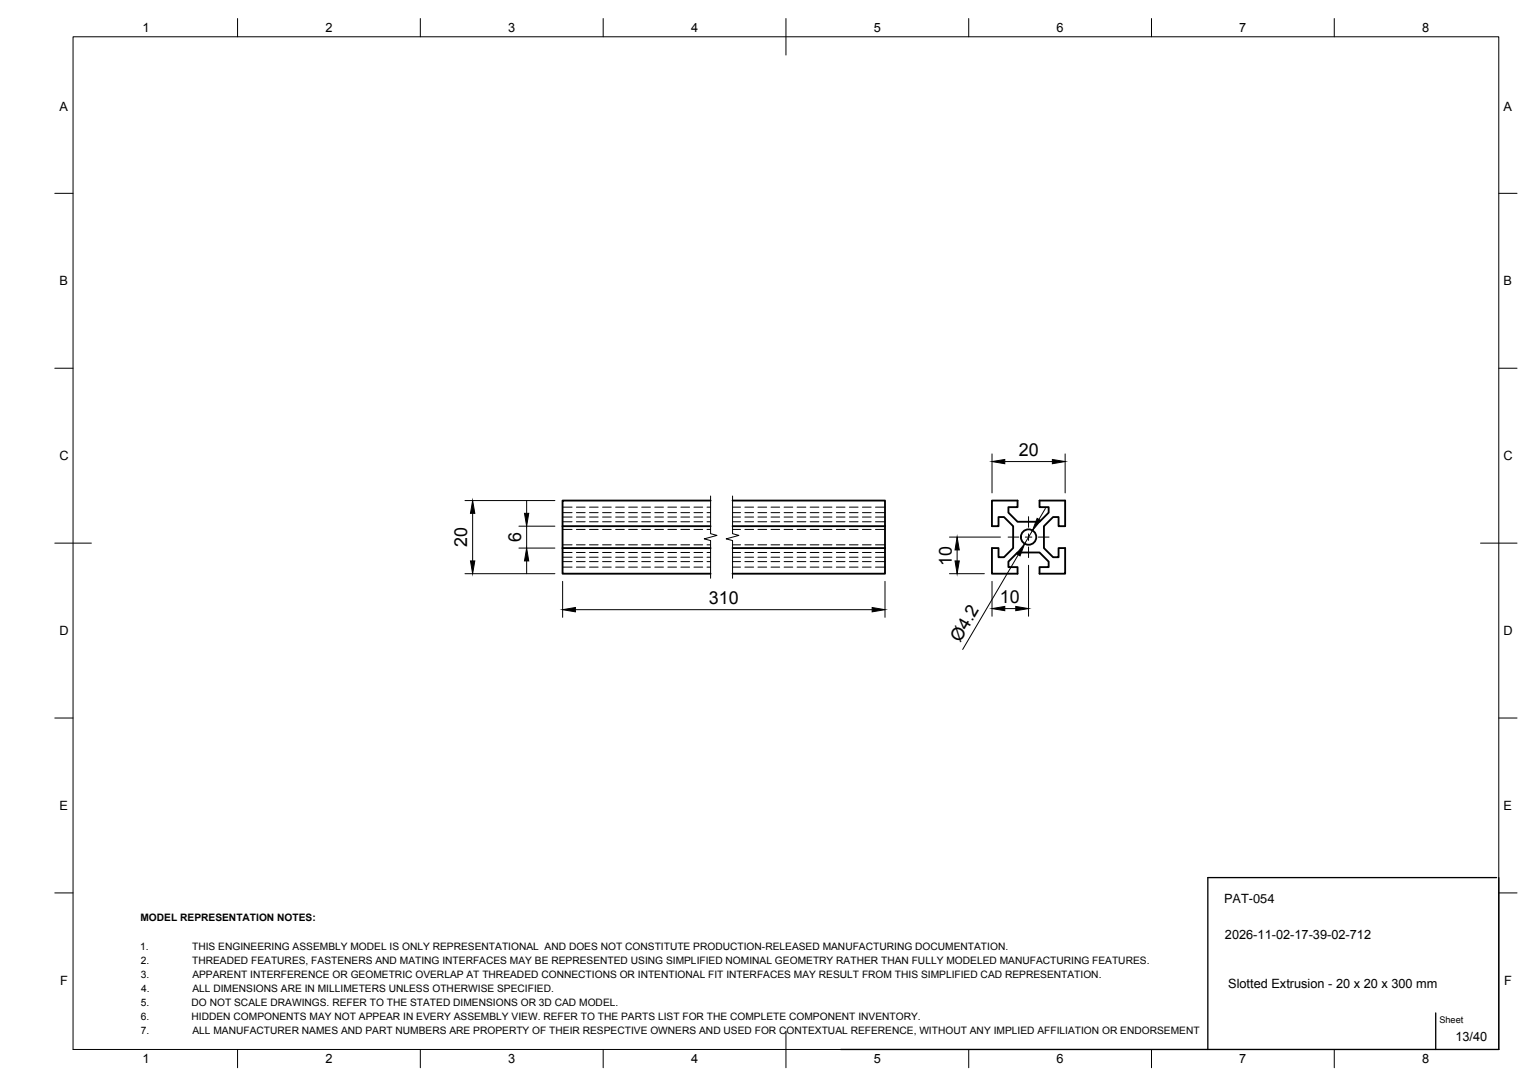
ISO-10303-21;
HEADER;
/* Generated by software containing ST-Developer
 * from STEP Tools, Inc. (www.steptools.com) 
 */

FILE_DESCRIPTION(
/* description */ ('PAT-054'),
/* implementation_level */ '2;1');

FILE_NAME(
/* name */ 'Slotted Extrusion - 20 x 20 x 300 mm.step',
/* time_stamp */ '2026-10-29T16:38:13-07:00',
/* author */ (''),
/* organization */ (''),
/* preprocessor_version */ 'ST-DEVELOPER v20.2',
/* originating_system */ 'Autodesk Translation Framework v15.17.0.0',
/* authorisation */ '');

FILE_SCHEMA (('AUTOMOTIVE_DESIGN { 1 0 10303 214 3 1 1 }'));
ENDSEC;

DATA;
#10=MECHANICAL_DESIGN_GEOMETRIC_PRESENTATION_REPRESENTATION('',(#933),#33981);
#830=SHAPE_REPRESENTATION_RELATIONSHIP('SRR','None',#34205,#874);
#874=ADVANCED_BREP_SHAPE_REPRESENTATION('',(#992),#33953);
#933=STYLED_ITEM('',(#34531),#992);
#992=MANIFOLD_SOLID_BREP('Body1',#13044);
#1146=FACE_BOUND('',#2730,.T.);
#1147=FACE_BOUND('',#2732,.T.);
#1344=PLANE('',#14134);
#1345=PLANE('',#14135);
#1346=PLANE('',#14136);
#1347=PLANE('',#14137);
#1348=PLANE('',#14138);
#1349=PLANE('',#14139);
#1350=PLANE('',#14140);
#1351=PLANE('',#14141);
#1352=PLANE('',#14142);
#1353=PLANE('',#14143);
#1354=PLANE('',#14144);
#1355=PLANE('',#14145);
#1356=PLANE('',#14146);
#1357=PLANE('',#14147);
#1358=PLANE('',#14148);
#1359=PLANE('',#14149);
#1360=PLANE('',#14150);
#1361=PLANE('',#14151);
#1362=PLANE('',#14152);
#1363=PLANE('',#14153);
#1364=PLANE('',#14154);
#1365=PLANE('',#14155);
#1366=PLANE('',#14156);
#1367=PLANE('',#14157);
#1368=PLANE('',#14158);
#1369=PLANE('',#14159);
#1370=PLANE('',#14160);
#1371=PLANE('',#14161);
#1372=PLANE('',#14162);
#1373=PLANE('',#14163);
#1374=PLANE('',#14164);
#1375=PLANE('',#14165);
#1376=PLANE('',#14166);
#1377=PLANE('',#14167);
#1378=PLANE('',#14168);
#1379=PLANE('',#14169);
#1380=PLANE('',#14173);
#1381=PLANE('',#14174);
#1382=PLANE('',#14175);
#1383=PLANE('',#14176);
#1384=PLANE('',#14177);
#1385=PLANE('',#14178);
#1386=PLANE('',#14179);
#1387=PLANE('',#14180);
#1388=PLANE('',#14181);
#1389=PLANE('',#14182);
#1827=FACE_OUTER_BOUND('',#2684,.T.);
#1828=FACE_OUTER_BOUND('',#2685,.T.);
#1829=FACE_OUTER_BOUND('',#2686,.T.);
#1830=FACE_OUTER_BOUND('',#2687,.T.);
#1831=FACE_OUTER_BOUND('',#2688,.T.);
#1832=FACE_OUTER_BOUND('',#2689,.T.);
#1833=FACE_OUTER_BOUND('',#2690,.T.);
#1834=FACE_OUTER_BOUND('',#2691,.T.);
#1835=FACE_OUTER_BOUND('',#2692,.T.);
#1836=FACE_OUTER_BOUND('',#2693,.T.);
#1837=FACE_OUTER_BOUND('',#2694,.T.);
#1838=FACE_OUTER_BOUND('',#2695,.T.);
#1839=FACE_OUTER_BOUND('',#2696,.T.);
#1840=FACE_OUTER_BOUND('',#2697,.T.);
#1841=FACE_OUTER_BOUND('',#2698,.T.);
#1842=FACE_OUTER_BOUND('',#2699,.T.);
#1843=FACE_OUTER_BOUND('',#2700,.T.);
#1844=FACE_OUTER_BOUND('',#2701,.T.);
#1845=FACE_OUTER_BOUND('',#2702,.T.);
#1846=FACE_OUTER_BOUND('',#2703,.T.);
#1847=FACE_OUTER_BOUND('',#2704,.T.);
#1848=FACE_OUTER_BOUND('',#2705,.T.);
#1849=FACE_OUTER_BOUND('',#2706,.T.);
#1850=FACE_OUTER_BOUND('',#2707,.T.);
#1851=FACE_OUTER_BOUND('',#2708,.T.);
#1852=FACE_OUTER_BOUND('',#2709,.T.);
#1853=FACE_OUTER_BOUND('',#2710,.T.);
#1854=FACE_OUTER_BOUND('',#2711,.T.);
#1855=FACE_OUTER_BOUND('',#2712,.T.);
#1856=FACE_OUTER_BOUND('',#2713,.T.);
#1857=FACE_OUTER_BOUND('',#2714,.T.);
#1858=FACE_OUTER_BOUND('',#2715,.T.);
#1859=FACE_OUTER_BOUND('',#2716,.T.);
#1860=FACE_OUTER_BOUND('',#2717,.T.);
#1861=FACE_OUTER_BOUND('',#2718,.T.);
#1862=FACE_OUTER_BOUND('',#2719,.T.);
#1863=FACE_OUTER_BOUND('',#2720,.T.);
#1864=FACE_OUTER_BOUND('',#2721,.T.);
#1865=FACE_OUTER_BOUND('',#2722,.T.);
#1866=FACE_OUTER_BOUND('',#2723,.T.);
#1867=FACE_OUTER_BOUND('',#2724,.T.);
#1868=FACE_OUTER_BOUND('',#2725,.T.);
#1869=FACE_OUTER_BOUND('',#2726,.T.);
#1870=FACE_OUTER_BOUND('',#2727,.T.);
#1871=FACE_OUTER_BOUND('',#2728,.T.);
#1872=FACE_OUTER_BOUND('',#2729,.T.);
#1873=FACE_OUTER_BOUND('',#2731,.T.);
#2684=EDGE_LOOP('',(#9637,#9638,#9639,#9640));
#2685=EDGE_LOOP('',(#9641,#9642,#9643,#9644));
#2686=EDGE_LOOP('',(#9645,#9646,#9647,#9648));
#2687=EDGE_LOOP('',(#9649,#9650,#9651,#9652));
#2688=EDGE_LOOP('',(#9653,#9654,#9655,#9656));
#2689=EDGE_LOOP('',(#9657,#9658,#9659,#9660));
#2690=EDGE_LOOP('',(#9661,#9662,#9663,#9664));
#2691=EDGE_LOOP('',(#9665,#9666,#9667,#9668));
#2692=EDGE_LOOP('',(#9669,#9670,#9671,#9672));
#2693=EDGE_LOOP('',(#9673,#9674,#9675,#9676));
#2694=EDGE_LOOP('',(#9677,#9678,#9679,#9680));
#2695=EDGE_LOOP('',(#9681,#9682,#9683,#9684));
#2696=EDGE_LOOP('',(#9685,#9686,#9687,#9688));
#2697=EDGE_LOOP('',(#9689,#9690,#9691,#9692));
#2698=EDGE_LOOP('',(#9693,#9694,#9695,#9696));
#2699=EDGE_LOOP('',(#9697,#9698,#9699,#9700));
#2700=EDGE_LOOP('',(#9701,#9702,#9703,#9704));
#2701=EDGE_LOOP('',(#9705,#9706,#9707,#9708));
#2702=EDGE_LOOP('',(#9709,#9710,#9711,#9712));
#2703=EDGE_LOOP('',(#9713,#9714,#9715,#9716));
#2704=EDGE_LOOP('',(#9717,#9718,#9719,#9720));
#2705=EDGE_LOOP('',(#9721,#9722,#9723,#9724));
#2706=EDGE_LOOP('',(#9725,#9726,#9727,#9728));
#2707=EDGE_LOOP('',(#9729,#9730,#9731,#9732));
#2708=EDGE_LOOP('',(#9733,#9734,#9735,#9736));
#2709=EDGE_LOOP('',(#9737,#9738,#9739,#9740));
#2710=EDGE_LOOP('',(#9741,#9742,#9743,#9744));
#2711=EDGE_LOOP('',(#9745,#9746,#9747,#9748));
#2712=EDGE_LOOP('',(#9749,#9750,#9751,#9752));
#2713=EDGE_LOOP('',(#9753,#9754,#9755,#9756));
#2714=EDGE_LOOP('',(#9757,#9758,#9759,#9760));
#2715=EDGE_LOOP('',(#9761,#9762,#9763,#9764));
#2716=EDGE_LOOP('',(#9765,#9766,#9767,#9768));
#2717=EDGE_LOOP('',(#9769,#9770,#9771,#9772));
#2718=EDGE_LOOP('',(#9773,#9774,#9775,#9776));
#2719=EDGE_LOOP('',(#9777,#9778,#9779,#9780));
#2720=EDGE_LOOP('',(#9781,#9782,#9783,#9784));
#2721=EDGE_LOOP('',(#9785,#9786,#9787,#9788));
#2722=EDGE_LOOP('',(#9789,#9790,#9791,#9792));
#2723=EDGE_LOOP('',(#9793,#9794,#9795,#9796));
#2724=EDGE_LOOP('',(#9797,#9798,#9799,#9800));
#2725=EDGE_LOOP('',(#9801,#9802,#9803,#9804));
#2726=EDGE_LOOP('',(#9805,#9806,#9807,#9808));
#2727=EDGE_LOOP('',(#9809,#9810,#9811,#9812));
#2728=EDGE_LOOP('',(#9813,#9814,#9815,#9816));
#2729=EDGE_LOOP('',(#9817,#9818,#9819,#9820,#9821,#9822,#9823,#9824,#9825,
#9826,#9827,#9828,#9829,#9830,#9831,#9832,#9833,#9834,#9835,#9836,#9837,
#9838,#9839,#9840,#9841,#9842,#9843,#9844,#9845,#9846,#9847,#9848,#9849,
#9850,#9851,#9852,#9853,#9854,#9855,#9856,#9857,#9858,#9859,#9860));
#2730=EDGE_LOOP('',(#9861));
#2731=EDGE_LOOP('',(#9862,#9863,#9864,#9865,#9866,#9867,#9868,#9869,#9870,
#9871,#9872,#9873,#9874,#9875,#9876,#9877,#9878,#9879,#9880,#9881,#9882,
#9883,#9884,#9885,#9886,#9887,#9888,#9889,#9890,#9891,#9892,#9893,#9894,
#9895,#9896,#9897,#9898,#9899,#9900,#9901,#9902,#9903,#9904,#9905));
#2732=EDGE_LOOP('',(#9906));
#3490=LINE('',#20381,#4424);
#3491=LINE('',#20383,#4425);
#3492=LINE('',#20385,#4426);
#3493=LINE('',#20386,#4427);
#3494=LINE('',#20389,#4428);
#3495=LINE('',#20391,#4429);
#3496=LINE('',#20392,#4430);
#3497=LINE('',#20395,#4431);
#3498=LINE('',#20397,#4432);
#3499=LINE('',#20398,#4433);
#3500=LINE('',#20401,#4434);
#3501=LINE('',#20403,#4435);
#3502=LINE('',#20404,#4436);
#3503=LINE('',#20407,#4437);
#3504=LINE('',#20409,#4438);
#3505=LINE('',#20410,#4439);
#3506=LINE('',#20413,#4440);
#3507=LINE('',#20415,#4441);
#3508=LINE('',#20416,#4442);
#3509=LINE('',#20419,#4443);
#3510=LINE('',#20421,#4444);
#3511=LINE('',#20422,#4445);
#3512=LINE('',#20425,#4446);
#3513=LINE('',#20427,#4447);
#3514=LINE('',#20428,#4448);
#3515=LINE('',#20431,#4449);
#3516=LINE('',#20433,#4450);
#3517=LINE('',#20434,#4451);
#3518=LINE('',#20438,#4452);
#3519=LINE('',#20440,#4453);
#3520=LINE('',#20442,#4454);
#3521=LINE('',#20443,#4455);
#3522=LINE('',#20446,#4456);
#3523=LINE('',#20448,#4457);
#3524=LINE('',#20449,#4458);
#3525=LINE('',#20452,#4459);
#3526=LINE('',#20454,#4460);
#3527=LINE('',#20455,#4461);
#3528=LINE('',#20458,#4462);
#3529=LINE('',#20460,#4463);
#3530=LINE('',#20461,#4464);
#3531=LINE('',#20464,#4465);
#3532=LINE('',#20466,#4466);
#3533=LINE('',#20467,#4467);
#3534=LINE('',#20470,#4468);
#3535=LINE('',#20472,#4469);
#3536=LINE('',#20473,#4470);
#3537=LINE('',#20476,#4471);
#3538=LINE('',#20478,#4472);
#3539=LINE('',#20479,#4473);
#3540=LINE('',#20482,#4474);
#3541=LINE('',#20484,#4475);
#3542=LINE('',#20485,#4476);
#3543=LINE('',#20488,#4477);
#3544=LINE('',#20490,#4478);
#3545=LINE('',#20491,#4479);
#3546=LINE('',#20495,#4480);
#3547=LINE('',#20497,#4481);
#3548=LINE('',#20499,#4482);
#3549=LINE('',#20500,#4483);
#3550=LINE('',#20503,#4484);
#3551=LINE('',#20505,#4485);
#3552=LINE('',#20506,#4486);
#3553=LINE('',#20509,#4487);
#3554=LINE('',#20511,#4488);
#3555=LINE('',#20512,#4489);
#3556=LINE('',#20515,#4490);
#3557=LINE('',#20517,#4491);
#3558=LINE('',#20518,#4492);
#3559=LINE('',#20521,#4493);
#3560=LINE('',#20523,#4494);
#3561=LINE('',#20524,#4495);
#3562=LINE('',#20527,#4496);
#3563=LINE('',#20529,#4497);
#3564=LINE('',#20530,#4498);
#3565=LINE('',#20533,#4499);
#3566=LINE('',#20535,#4500);
#3567=LINE('',#20536,#4501);
#3568=LINE('',#20539,#4502);
#3569=LINE('',#20541,#4503);
#3570=LINE('',#20542,#4504);
#3571=LINE('',#20545,#4505);
#3572=LINE('',#20547,#4506);
#3573=LINE('',#20548,#4507);
#3574=LINE('',#20552,#4508);
#3575=LINE('',#20554,#4509);
#3576=LINE('',#20556,#4510);
#3577=LINE('',#20557,#4511);
#3578=LINE('',#20560,#4512);
#3579=LINE('',#20562,#4513);
#3580=LINE('',#20563,#4514);
#3581=LINE('',#20566,#4515);
#3582=LINE('',#20568,#4516);
#3583=LINE('',#20569,#4517);
#3584=LINE('',#20572,#4518);
#3585=LINE('',#20574,#4519);
#3586=LINE('',#20575,#4520);
#3587=LINE('',#20578,#4521);
#3588=LINE('',#20580,#4522);
#3589=LINE('',#20581,#4523);
#3590=LINE('',#20584,#4524);
#3591=LINE('',#20586,#4525);
#3592=LINE('',#20587,#4526);
#3593=LINE('',#20590,#4527);
#3594=LINE('',#20592,#4528);
#3595=LINE('',#20593,#4529);
#3596=LINE('',#20596,#4530);
#3597=LINE('',#20598,#4531);
#3598=LINE('',#20599,#4532);
#3599=LINE('',#20602,#4533);
#3600=LINE('',#20604,#4534);
#3601=LINE('',#20605,#4535);
#3602=LINE('',#20610,#4536);
#3603=LINE('',#20614,#4537);
#3604=LINE('',#20616,#4538);
#3605=LINE('',#20617,#4539);
#3606=LINE('',#20620,#4540);
#3607=LINE('',#20622,#4541);
#3608=LINE('',#20623,#4542);
#3609=LINE('',#20625,#4543);
#3610=LINE('',#20626,#4544);
#3611=LINE('',#20629,#4545);
#3612=LINE('',#20631,#4546);
#3613=LINE('',#20632,#4547);
#3614=LINE('',#20634,#4548);
#3615=LINE('',#20635,#4549);
#3616=LINE('',#20638,#4550);
#3617=LINE('',#20640,#4551);
#3618=LINE('',#20641,#4552);
#3619=LINE('',#20643,#4553);
#3620=LINE('',#20644,#4554);
#3621=LINE('',#20646,#4555);
#3622=LINE('',#20647,#4556);
#4424=VECTOR('',#16295,1.);
#4425=VECTOR('',#16296,1.);
#4426=VECTOR('',#16297,1.);
#4427=VECTOR('',#16298,1.);
#4428=VECTOR('',#16301,1.);
#4429=VECTOR('',#16302,1.);
#4430=VECTOR('',#16303,1.);
#4431=VECTOR('',#16306,1.);
#4432=VECTOR('',#16307,1.);
#4433=VECTOR('',#16308,1.);
#4434=VECTOR('',#16311,1.);
#4435=VECTOR('',#16312,1.);
#4436=VECTOR('',#16313,1.);
#4437=VECTOR('',#16316,1.);
#4438=VECTOR('',#16317,1.);
#4439=VECTOR('',#16318,1.);
#4440=VECTOR('',#16321,1.);
#4441=VECTOR('',#16322,1.);
#4442=VECTOR('',#16323,1.);
#4443=VECTOR('',#16326,1.);
#4444=VECTOR('',#16327,1.);
#4445=VECTOR('',#16328,1.);
#4446=VECTOR('',#16331,1.);
#4447=VECTOR('',#16332,1.);
#4448=VECTOR('',#16333,1.);
#4449=VECTOR('',#16336,1.);
#4450=VECTOR('',#16337,1.);
#4451=VECTOR('',#16338,1.);
#4452=VECTOR('',#16341,1.);
#4453=VECTOR('',#16342,1.);
#4454=VECTOR('',#16343,1.);
#4455=VECTOR('',#16344,1.);
#4456=VECTOR('',#16347,1.);
#4457=VECTOR('',#16348,1.);
#4458=VECTOR('',#16349,1.);
#4459=VECTOR('',#16352,1.);
#4460=VECTOR('',#16353,1.);
#4461=VECTOR('',#16354,1.);
#4462=VECTOR('',#16357,1.);
#4463=VECTOR('',#16358,1.);
#4464=VECTOR('',#16359,1.);
#4465=VECTOR('',#16362,1.);
#4466=VECTOR('',#16363,1.);
#4467=VECTOR('',#16364,1.);
#4468=VECTOR('',#16367,1.);
#4469=VECTOR('',#16368,1.);
#4470=VECTOR('',#16369,1.);
#4471=VECTOR('',#16372,1.);
#4472=VECTOR('',#16373,1.);
#4473=VECTOR('',#16374,1.);
#4474=VECTOR('',#16377,1.);
#4475=VECTOR('',#16378,1.);
#4476=VECTOR('',#16379,1.);
#4477=VECTOR('',#16382,1.);
#4478=VECTOR('',#16383,1.);
#4479=VECTOR('',#16384,1.);
#4480=VECTOR('',#16387,1.);
#4481=VECTOR('',#16388,1.);
#4482=VECTOR('',#16389,1.);
#4483=VECTOR('',#16390,1.);
#4484=VECTOR('',#16393,1.);
#4485=VECTOR('',#16394,1.);
#4486=VECTOR('',#16395,1.);
#4487=VECTOR('',#16398,1.);
#4488=VECTOR('',#16399,1.);
#4489=VECTOR('',#16400,1.);
#4490=VECTOR('',#16403,1.);
#4491=VECTOR('',#16404,1.);
#4492=VECTOR('',#16405,1.);
#4493=VECTOR('',#16408,1.);
#4494=VECTOR('',#16409,1.);
#4495=VECTOR('',#16410,1.);
#4496=VECTOR('',#16413,1.);
#4497=VECTOR('',#16414,1.);
#4498=VECTOR('',#16415,1.);
#4499=VECTOR('',#16418,1.);
#4500=VECTOR('',#16419,1.);
#4501=VECTOR('',#16420,1.);
#4502=VECTOR('',#16423,1.);
#4503=VECTOR('',#16424,1.);
#4504=VECTOR('',#16425,1.);
#4505=VECTOR('',#16428,1.);
#4506=VECTOR('',#16429,1.);
#4507=VECTOR('',#16430,1.);
#4508=VECTOR('',#16433,1.);
#4509=VECTOR('',#16434,1.);
#4510=VECTOR('',#16435,1.);
#4511=VECTOR('',#16436,1.);
#4512=VECTOR('',#16439,1.);
#4513=VECTOR('',#16440,1.);
#4514=VECTOR('',#16441,1.);
#4515=VECTOR('',#16444,1.);
#4516=VECTOR('',#16445,1.);
#4517=VECTOR('',#16446,1.);
#4518=VECTOR('',#16449,1.);
#4519=VECTOR('',#16450,1.);
#4520=VECTOR('',#16451,1.);
#4521=VECTOR('',#16454,1.);
#4522=VECTOR('',#16455,1.);
#4523=VECTOR('',#16456,1.);
#4524=VECTOR('',#16459,1.);
#4525=VECTOR('',#16460,1.);
#4526=VECTOR('',#16461,1.);
#4527=VECTOR('',#16464,1.);
#4528=VECTOR('',#16465,1.);
#4529=VECTOR('',#16466,1.);
#4530=VECTOR('',#16469,1.);
#4531=VECTOR('',#16470,1.);
#4532=VECTOR('',#16471,1.);
#4533=VECTOR('',#16474,1.);
#4534=VECTOR('',#16475,1.);
#4535=VECTOR('',#16476,1.);
#4536=VECTOR('',#16481,0.21);
#4537=VECTOR('',#16486,1.);
#4538=VECTOR('',#16487,1.);
#4539=VECTOR('',#16488,1.);
#4540=VECTOR('',#16491,1.);
#4541=VECTOR('',#16492,1.);
#4542=VECTOR('',#16493,1.);
#4543=VECTOR('',#16496,1.);
#4544=VECTOR('',#16497,1.);
#4545=VECTOR('',#16500,1.);
#4546=VECTOR('',#16501,1.);
#4547=VECTOR('',#16502,1.);
#4548=VECTOR('',#16505,1.);
#4549=VECTOR('',#16506,1.);
#4550=VECTOR('',#16509,1.);
#4551=VECTOR('',#16510,1.);
#4552=VECTOR('',#16511,1.);
#4553=VECTOR('',#16514,1.);
#4554=VECTOR('',#16515,1.);
#4555=VECTOR('',#16518,1.);
#4556=VECTOR('',#16519,1.);
#5394=CIRCLE('',#14171,0.21);
#5395=CIRCLE('',#14172,0.21);
#5970=VERTEX_POINT('',#20379);
#5971=VERTEX_POINT('',#20380);
#5972=VERTEX_POINT('',#20382);
#5973=VERTEX_POINT('',#20384);
#5974=VERTEX_POINT('',#20388);
#5975=VERTEX_POINT('',#20390);
#5976=VERTEX_POINT('',#20394);
#5977=VERTEX_POINT('',#20396);
#5978=VERTEX_POINT('',#20400);
#5979=VERTEX_POINT('',#20402);
#5980=VERTEX_POINT('',#20406);
#5981=VERTEX_POINT('',#20408);
#5982=VERTEX_POINT('',#20412);
#5983=VERTEX_POINT('',#20414);
#5984=VERTEX_POINT('',#20418);
#5985=VERTEX_POINT('',#20420);
#5986=VERTEX_POINT('',#20424);
#5987=VERTEX_POINT('',#20426);
#5988=VERTEX_POINT('',#20430);
#5989=VERTEX_POINT('',#20432);
#5990=VERTEX_POINT('',#20436);
#5991=VERTEX_POINT('',#20437);
#5992=VERTEX_POINT('',#20439);
#5993=VERTEX_POINT('',#20441);
#5994=VERTEX_POINT('',#20445);
#5995=VERTEX_POINT('',#20447);
#5996=VERTEX_POINT('',#20451);
#5997=VERTEX_POINT('',#20453);
#5998=VERTEX_POINT('',#20457);
#5999=VERTEX_POINT('',#20459);
#6000=VERTEX_POINT('',#20463);
#6001=VERTEX_POINT('',#20465);
#6002=VERTEX_POINT('',#20469);
#6003=VERTEX_POINT('',#20471);
#6004=VERTEX_POINT('',#20475);
#6005=VERTEX_POINT('',#20477);
#6006=VERTEX_POINT('',#20481);
#6007=VERTEX_POINT('',#20483);
#6008=VERTEX_POINT('',#20487);
#6009=VERTEX_POINT('',#20489);
#6010=VERTEX_POINT('',#20493);
#6011=VERTEX_POINT('',#20494);
#6012=VERTEX_POINT('',#20496);
#6013=VERTEX_POINT('',#20498);
#6014=VERTEX_POINT('',#20502);
#6015=VERTEX_POINT('',#20504);
#6016=VERTEX_POINT('',#20508);
#6017=VERTEX_POINT('',#20510);
#6018=VERTEX_POINT('',#20514);
#6019=VERTEX_POINT('',#20516);
#6020=VERTEX_POINT('',#20520);
#6021=VERTEX_POINT('',#20522);
#6022=VERTEX_POINT('',#20526);
#6023=VERTEX_POINT('',#20528);
#6024=VERTEX_POINT('',#20532);
#6025=VERTEX_POINT('',#20534);
#6026=VERTEX_POINT('',#20538);
#6027=VERTEX_POINT('',#20540);
#6028=VERTEX_POINT('',#20544);
#6029=VERTEX_POINT('',#20546);
#6030=VERTEX_POINT('',#20550);
#6031=VERTEX_POINT('',#20551);
#6032=VERTEX_POINT('',#20553);
#6033=VERTEX_POINT('',#20555);
#6034=VERTEX_POINT('',#20559);
#6035=VERTEX_POINT('',#20561);
#6036=VERTEX_POINT('',#20565);
#6037=VERTEX_POINT('',#20567);
#6038=VERTEX_POINT('',#20571);
#6039=VERTEX_POINT('',#20573);
#6040=VERTEX_POINT('',#20577);
#6041=VERTEX_POINT('',#20579);
#6042=VERTEX_POINT('',#20583);
#6043=VERTEX_POINT('',#20585);
#6044=VERTEX_POINT('',#20589);
#6045=VERTEX_POINT('',#20591);
#6046=VERTEX_POINT('',#20595);
#6047=VERTEX_POINT('',#20597);
#6048=VERTEX_POINT('',#20601);
#6049=VERTEX_POINT('',#20603);
#6050=VERTEX_POINT('',#20607);
#6051=VERTEX_POINT('',#20609);
#6052=VERTEX_POINT('',#20613);
#6053=VERTEX_POINT('',#20615);
#6054=VERTEX_POINT('',#20619);
#6055=VERTEX_POINT('',#20621);
#6056=VERTEX_POINT('',#20628);
#6057=VERTEX_POINT('',#20630);
#6058=VERTEX_POINT('',#20637);
#6059=VERTEX_POINT('',#20639);
#7318=EDGE_CURVE('',#5970,#5971,#3490,.T.);
#7319=EDGE_CURVE('',#5970,#5972,#3491,.T.);
#7320=EDGE_CURVE('',#5973,#5972,#3492,.T.);
#7321=EDGE_CURVE('',#5971,#5973,#3493,.T.);
#7322=EDGE_CURVE('',#5974,#5970,#3494,.T.);
#7323=EDGE_CURVE('',#5974,#5975,#3495,.T.);
#7324=EDGE_CURVE('',#5972,#5975,#3496,.T.);
#7325=EDGE_CURVE('',#5976,#5974,#3497,.T.);
#7326=EDGE_CURVE('',#5976,#5977,#3498,.T.);
#7327=EDGE_CURVE('',#5975,#5977,#3499,.T.);
#7328=EDGE_CURVE('',#5978,#5976,#3500,.T.);
#7329=EDGE_CURVE('',#5978,#5979,#3501,.T.);
#7330=EDGE_CURVE('',#5977,#5979,#3502,.T.);
#7331=EDGE_CURVE('',#5980,#5978,#3503,.T.);
#7332=EDGE_CURVE('',#5980,#5981,#3504,.T.);
#7333=EDGE_CURVE('',#5979,#5981,#3505,.T.);
#7334=EDGE_CURVE('',#5982,#5980,#3506,.T.);
#7335=EDGE_CURVE('',#5982,#5983,#3507,.T.);
#7336=EDGE_CURVE('',#5981,#5983,#3508,.T.);
#7337=EDGE_CURVE('',#5984,#5982,#3509,.T.);
#7338=EDGE_CURVE('',#5984,#5985,#3510,.T.);
#7339=EDGE_CURVE('',#5983,#5985,#3511,.T.);
#7340=EDGE_CURVE('',#5986,#5984,#3512,.T.);
#7341=EDGE_CURVE('',#5986,#5987,#3513,.T.);
#7342=EDGE_CURVE('',#5985,#5987,#3514,.T.);
#7343=EDGE_CURVE('',#5988,#5986,#3515,.T.);
#7344=EDGE_CURVE('',#5989,#5988,#3516,.T.);
#7345=EDGE_CURVE('',#5987,#5989,#3517,.T.);
#7346=EDGE_CURVE('',#5990,#5991,#3518,.T.);
#7347=EDGE_CURVE('',#5990,#5992,#3519,.T.);
#7348=EDGE_CURVE('',#5993,#5992,#3520,.T.);
#7349=EDGE_CURVE('',#5991,#5993,#3521,.T.);
#7350=EDGE_CURVE('',#5994,#5990,#3522,.T.);
#7351=EDGE_CURVE('',#5994,#5995,#3523,.T.);
#7352=EDGE_CURVE('',#5992,#5995,#3524,.T.);
#7353=EDGE_CURVE('',#5996,#5994,#3525,.T.);
#7354=EDGE_CURVE('',#5996,#5997,#3526,.T.);
#7355=EDGE_CURVE('',#5995,#5997,#3527,.T.);
#7356=EDGE_CURVE('',#5998,#5996,#3528,.T.);
#7357=EDGE_CURVE('',#5998,#5999,#3529,.T.);
#7358=EDGE_CURVE('',#5997,#5999,#3530,.T.);
#7359=EDGE_CURVE('',#6000,#5998,#3531,.T.);
#7360=EDGE_CURVE('',#6000,#6001,#3532,.T.);
#7361=EDGE_CURVE('',#5999,#6001,#3533,.T.);
#7362=EDGE_CURVE('',#6002,#6000,#3534,.T.);
#7363=EDGE_CURVE('',#6002,#6003,#3535,.T.);
#7364=EDGE_CURVE('',#6001,#6003,#3536,.T.);
#7365=EDGE_CURVE('',#6004,#6002,#3537,.T.);
#7366=EDGE_CURVE('',#6004,#6005,#3538,.T.);
#7367=EDGE_CURVE('',#6003,#6005,#3539,.T.);
#7368=EDGE_CURVE('',#6006,#6004,#3540,.T.);
#7369=EDGE_CURVE('',#6006,#6007,#3541,.T.);
#7370=EDGE_CURVE('',#6005,#6007,#3542,.T.);
#7371=EDGE_CURVE('',#6008,#6006,#3543,.T.);
#7372=EDGE_CURVE('',#6009,#6008,#3544,.T.);
#7373=EDGE_CURVE('',#6007,#6009,#3545,.T.);
#7374=EDGE_CURVE('',#6010,#6011,#3546,.T.);
#7375=EDGE_CURVE('',#6010,#6012,#3547,.T.);
#7376=EDGE_CURVE('',#6013,#6012,#3548,.T.);
#7377=EDGE_CURVE('',#6011,#6013,#3549,.T.);
#7378=EDGE_CURVE('',#6014,#6010,#3550,.T.);
#7379=EDGE_CURVE('',#6014,#6015,#3551,.T.);
#7380=EDGE_CURVE('',#6012,#6015,#3552,.T.);
#7381=EDGE_CURVE('',#6016,#6014,#3553,.T.);
#7382=EDGE_CURVE('',#6016,#6017,#3554,.T.);
#7383=EDGE_CURVE('',#6015,#6017,#3555,.T.);
#7384=EDGE_CURVE('',#6018,#6016,#3556,.T.);
#7385=EDGE_CURVE('',#6018,#6019,#3557,.T.);
#7386=EDGE_CURVE('',#6017,#6019,#3558,.T.);
#7387=EDGE_CURVE('',#6020,#6018,#3559,.T.);
#7388=EDGE_CURVE('',#6020,#6021,#3560,.T.);
#7389=EDGE_CURVE('',#6019,#6021,#3561,.T.);
#7390=EDGE_CURVE('',#6022,#6020,#3562,.T.);
#7391=EDGE_CURVE('',#6022,#6023,#3563,.T.);
#7392=EDGE_CURVE('',#6021,#6023,#3564,.T.);
#7393=EDGE_CURVE('',#6024,#6022,#3565,.T.);
#7394=EDGE_CURVE('',#6024,#6025,#3566,.T.);
#7395=EDGE_CURVE('',#6023,#6025,#3567,.T.);
#7396=EDGE_CURVE('',#6026,#6024,#3568,.T.);
#7397=EDGE_CURVE('',#6026,#6027,#3569,.T.);
#7398=EDGE_CURVE('',#6025,#6027,#3570,.T.);
#7399=EDGE_CURVE('',#6028,#6026,#3571,.T.);
#7400=EDGE_CURVE('',#6029,#6028,#3572,.T.);
#7401=EDGE_CURVE('',#6027,#6029,#3573,.T.);
#7402=EDGE_CURVE('',#6030,#6031,#3574,.T.);
#7403=EDGE_CURVE('',#6030,#6032,#3575,.T.);
#7404=EDGE_CURVE('',#6033,#6032,#3576,.T.);
#7405=EDGE_CURVE('',#6031,#6033,#3577,.T.);
#7406=EDGE_CURVE('',#6034,#6030,#3578,.T.);
#7407=EDGE_CURVE('',#6034,#6035,#3579,.T.);
#7408=EDGE_CURVE('',#6032,#6035,#3580,.T.);
#7409=EDGE_CURVE('',#6036,#6034,#3581,.T.);
#7410=EDGE_CURVE('',#6036,#6037,#3582,.T.);
#7411=EDGE_CURVE('',#6035,#6037,#3583,.T.);
#7412=EDGE_CURVE('',#6038,#6036,#3584,.T.);
#7413=EDGE_CURVE('',#6038,#6039,#3585,.T.);
#7414=EDGE_CURVE('',#6037,#6039,#3586,.T.);
#7415=EDGE_CURVE('',#6040,#6038,#3587,.T.);
#7416=EDGE_CURVE('',#6040,#6041,#3588,.T.);
#7417=EDGE_CURVE('',#6039,#6041,#3589,.T.);
#7418=EDGE_CURVE('',#6042,#6040,#3590,.T.);
#7419=EDGE_CURVE('',#6042,#6043,#3591,.T.);
#7420=EDGE_CURVE('',#6041,#6043,#3592,.T.);
#7421=EDGE_CURVE('',#6044,#6042,#3593,.T.);
#7422=EDGE_CURVE('',#6044,#6045,#3594,.T.);
#7423=EDGE_CURVE('',#6043,#6045,#3595,.T.);
#7424=EDGE_CURVE('',#6046,#6044,#3596,.T.);
#7425=EDGE_CURVE('',#6046,#6047,#3597,.T.);
#7426=EDGE_CURVE('',#6045,#6047,#3598,.T.);
#7427=EDGE_CURVE('',#6048,#6046,#3599,.T.);
#7428=EDGE_CURVE('',#6049,#6048,#3600,.T.);
#7429=EDGE_CURVE('',#6047,#6049,#3601,.T.);
#7430=EDGE_CURVE('',#6050,#6050,#5394,.T.);
#7431=EDGE_CURVE('',#6050,#6051,#3602,.T.);
#7432=EDGE_CURVE('',#6051,#6051,#5395,.T.);
#7433=EDGE_CURVE('',#5988,#6052,#3603,.T.);
#7434=EDGE_CURVE('',#6052,#6053,#3604,.T.);
#7435=EDGE_CURVE('',#5989,#6053,#3605,.T.);
#7436=EDGE_CURVE('',#6054,#5973,#3606,.T.);
#7437=EDGE_CURVE('',#6055,#6054,#3607,.T.);
#7438=EDGE_CURVE('',#6055,#5971,#3608,.T.);
#7439=EDGE_CURVE('',#6008,#6055,#3609,.T.);
#7440=EDGE_CURVE('',#6009,#6054,#3610,.T.);
#7441=EDGE_CURVE('',#6056,#5993,#3611,.T.);
#7442=EDGE_CURVE('',#6057,#6056,#3612,.T.);
#7443=EDGE_CURVE('',#6057,#5991,#3613,.T.);
#7444=EDGE_CURVE('',#6028,#6057,#3614,.T.);
#7445=EDGE_CURVE('',#6029,#6056,#3615,.T.);
#7446=EDGE_CURVE('',#6058,#6013,#3616,.T.);
#7447=EDGE_CURVE('',#6059,#6058,#3617,.T.);
#7448=EDGE_CURVE('',#6059,#6011,#3618,.T.);
#7449=EDGE_CURVE('',#6048,#6059,#3619,.T.);
#7450=EDGE_CURVE('',#6049,#6058,#3620,.T.);
#7451=EDGE_CURVE('',#6053,#6033,#3621,.T.);
#7452=EDGE_CURVE('',#6052,#6031,#3622,.T.);
#9637=ORIENTED_EDGE('',*,*,#7318,.F.);
#9638=ORIENTED_EDGE('',*,*,#7319,.T.);
#9639=ORIENTED_EDGE('',*,*,#7320,.F.);
#9640=ORIENTED_EDGE('',*,*,#7321,.F.);
#9641=ORIENTED_EDGE('',*,*,#7322,.F.);
#9642=ORIENTED_EDGE('',*,*,#7323,.T.);
#9643=ORIENTED_EDGE('',*,*,#7324,.F.);
#9644=ORIENTED_EDGE('',*,*,#7319,.F.);
#9645=ORIENTED_EDGE('',*,*,#7325,.F.);
#9646=ORIENTED_EDGE('',*,*,#7326,.T.);
#9647=ORIENTED_EDGE('',*,*,#7327,.F.);
#9648=ORIENTED_EDGE('',*,*,#7323,.F.);
#9649=ORIENTED_EDGE('',*,*,#7328,.F.);
#9650=ORIENTED_EDGE('',*,*,#7329,.T.);
#9651=ORIENTED_EDGE('',*,*,#7330,.F.);
#9652=ORIENTED_EDGE('',*,*,#7326,.F.);
#9653=ORIENTED_EDGE('',*,*,#7331,.F.);
#9654=ORIENTED_EDGE('',*,*,#7332,.T.);
#9655=ORIENTED_EDGE('',*,*,#7333,.F.);
#9656=ORIENTED_EDGE('',*,*,#7329,.F.);
#9657=ORIENTED_EDGE('',*,*,#7334,.F.);
#9658=ORIENTED_EDGE('',*,*,#7335,.T.);
#9659=ORIENTED_EDGE('',*,*,#7336,.F.);
#9660=ORIENTED_EDGE('',*,*,#7332,.F.);
#9661=ORIENTED_EDGE('',*,*,#7337,.F.);
#9662=ORIENTED_EDGE('',*,*,#7338,.T.);
#9663=ORIENTED_EDGE('',*,*,#7339,.F.);
#9664=ORIENTED_EDGE('',*,*,#7335,.F.);
#9665=ORIENTED_EDGE('',*,*,#7340,.F.);
#9666=ORIENTED_EDGE('',*,*,#7341,.T.);
#9667=ORIENTED_EDGE('',*,*,#7342,.F.);
#9668=ORIENTED_EDGE('',*,*,#7338,.F.);
#9669=ORIENTED_EDGE('',*,*,#7343,.F.);
#9670=ORIENTED_EDGE('',*,*,#7344,.F.);
#9671=ORIENTED_EDGE('',*,*,#7345,.F.);
#9672=ORIENTED_EDGE('',*,*,#7341,.F.);
#9673=ORIENTED_EDGE('',*,*,#7346,.F.);
#9674=ORIENTED_EDGE('',*,*,#7347,.T.);
#9675=ORIENTED_EDGE('',*,*,#7348,.F.);
#9676=ORIENTED_EDGE('',*,*,#7349,.F.);
#9677=ORIENTED_EDGE('',*,*,#7350,.F.);
#9678=ORIENTED_EDGE('',*,*,#7351,.T.);
#9679=ORIENTED_EDGE('',*,*,#7352,.F.);
#9680=ORIENTED_EDGE('',*,*,#7347,.F.);
#9681=ORIENTED_EDGE('',*,*,#7353,.F.);
#9682=ORIENTED_EDGE('',*,*,#7354,.T.);
#9683=ORIENTED_EDGE('',*,*,#7355,.F.);
#9684=ORIENTED_EDGE('',*,*,#7351,.F.);
#9685=ORIENTED_EDGE('',*,*,#7356,.F.);
#9686=ORIENTED_EDGE('',*,*,#7357,.T.);
#9687=ORIENTED_EDGE('',*,*,#7358,.F.);
#9688=ORIENTED_EDGE('',*,*,#7354,.F.);
#9689=ORIENTED_EDGE('',*,*,#7359,.F.);
#9690=ORIENTED_EDGE('',*,*,#7360,.T.);
#9691=ORIENTED_EDGE('',*,*,#7361,.F.);
#9692=ORIENTED_EDGE('',*,*,#7357,.F.);
#9693=ORIENTED_EDGE('',*,*,#7362,.F.);
#9694=ORIENTED_EDGE('',*,*,#7363,.T.);
#9695=ORIENTED_EDGE('',*,*,#7364,.F.);
#9696=ORIENTED_EDGE('',*,*,#7360,.F.);
#9697=ORIENTED_EDGE('',*,*,#7365,.F.);
#9698=ORIENTED_EDGE('',*,*,#7366,.T.);
#9699=ORIENTED_EDGE('',*,*,#7367,.F.);
#9700=ORIENTED_EDGE('',*,*,#7363,.F.);
#9701=ORIENTED_EDGE('',*,*,#7368,.F.);
#9702=ORIENTED_EDGE('',*,*,#7369,.T.);
#9703=ORIENTED_EDGE('',*,*,#7370,.F.);
#9704=ORIENTED_EDGE('',*,*,#7366,.F.);
#9705=ORIENTED_EDGE('',*,*,#7371,.F.);
#9706=ORIENTED_EDGE('',*,*,#7372,.F.);
#9707=ORIENTED_EDGE('',*,*,#7373,.F.);
#9708=ORIENTED_EDGE('',*,*,#7369,.F.);
#9709=ORIENTED_EDGE('',*,*,#7374,.F.);
#9710=ORIENTED_EDGE('',*,*,#7375,.T.);
#9711=ORIENTED_EDGE('',*,*,#7376,.F.);
#9712=ORIENTED_EDGE('',*,*,#7377,.F.);
#9713=ORIENTED_EDGE('',*,*,#7378,.F.);
#9714=ORIENTED_EDGE('',*,*,#7379,.T.);
#9715=ORIENTED_EDGE('',*,*,#7380,.F.);
#9716=ORIENTED_EDGE('',*,*,#7375,.F.);
#9717=ORIENTED_EDGE('',*,*,#7381,.F.);
#9718=ORIENTED_EDGE('',*,*,#7382,.T.);
#9719=ORIENTED_EDGE('',*,*,#7383,.F.);
#9720=ORIENTED_EDGE('',*,*,#7379,.F.);
#9721=ORIENTED_EDGE('',*,*,#7384,.F.);
#9722=ORIENTED_EDGE('',*,*,#7385,.T.);
#9723=ORIENTED_EDGE('',*,*,#7386,.F.);
#9724=ORIENTED_EDGE('',*,*,#7382,.F.);
#9725=ORIENTED_EDGE('',*,*,#7387,.F.);
#9726=ORIENTED_EDGE('',*,*,#7388,.T.);
#9727=ORIENTED_EDGE('',*,*,#7389,.F.);
#9728=ORIENTED_EDGE('',*,*,#7385,.F.);
#9729=ORIENTED_EDGE('',*,*,#7390,.F.);
#9730=ORIENTED_EDGE('',*,*,#7391,.T.);
#9731=ORIENTED_EDGE('',*,*,#7392,.F.);
#9732=ORIENTED_EDGE('',*,*,#7388,.F.);
#9733=ORIENTED_EDGE('',*,*,#7393,.F.);
#9734=ORIENTED_EDGE('',*,*,#7394,.T.);
#9735=ORIENTED_EDGE('',*,*,#7395,.F.);
#9736=ORIENTED_EDGE('',*,*,#7391,.F.);
#9737=ORIENTED_EDGE('',*,*,#7396,.F.);
#9738=ORIENTED_EDGE('',*,*,#7397,.T.);
#9739=ORIENTED_EDGE('',*,*,#7398,.F.);
#9740=ORIENTED_EDGE('',*,*,#7394,.F.);
#9741=ORIENTED_EDGE('',*,*,#7399,.F.);
#9742=ORIENTED_EDGE('',*,*,#7400,.F.);
#9743=ORIENTED_EDGE('',*,*,#7401,.F.);
#9744=ORIENTED_EDGE('',*,*,#7397,.F.);
#9745=ORIENTED_EDGE('',*,*,#7402,.F.);
#9746=ORIENTED_EDGE('',*,*,#7403,.T.);
#9747=ORIENTED_EDGE('',*,*,#7404,.F.);
#9748=ORIENTED_EDGE('',*,*,#7405,.F.);
#9749=ORIENTED_EDGE('',*,*,#7406,.F.);
#9750=ORIENTED_EDGE('',*,*,#7407,.T.);
#9751=ORIENTED_EDGE('',*,*,#7408,.F.);
#9752=ORIENTED_EDGE('',*,*,#7403,.F.);
#9753=ORIENTED_EDGE('',*,*,#7409,.F.);
#9754=ORIENTED_EDGE('',*,*,#7410,.T.);
#9755=ORIENTED_EDGE('',*,*,#7411,.F.);
#9756=ORIENTED_EDGE('',*,*,#7407,.F.);
#9757=ORIENTED_EDGE('',*,*,#7412,.F.);
#9758=ORIENTED_EDGE('',*,*,#7413,.T.);
#9759=ORIENTED_EDGE('',*,*,#7414,.F.);
#9760=ORIENTED_EDGE('',*,*,#7410,.F.);
#9761=ORIENTED_EDGE('',*,*,#7415,.F.);
#9762=ORIENTED_EDGE('',*,*,#7416,.T.);
#9763=ORIENTED_EDGE('',*,*,#7417,.F.);
#9764=ORIENTED_EDGE('',*,*,#7413,.F.);
#9765=ORIENTED_EDGE('',*,*,#7418,.F.);
#9766=ORIENTED_EDGE('',*,*,#7419,.T.);
#9767=ORIENTED_EDGE('',*,*,#7420,.F.);
#9768=ORIENTED_EDGE('',*,*,#7416,.F.);
#9769=ORIENTED_EDGE('',*,*,#7421,.F.);
#9770=ORIENTED_EDGE('',*,*,#7422,.T.);
#9771=ORIENTED_EDGE('',*,*,#7423,.F.);
#9772=ORIENTED_EDGE('',*,*,#7419,.F.);
#9773=ORIENTED_EDGE('',*,*,#7424,.F.);
#9774=ORIENTED_EDGE('',*,*,#7425,.T.);
#9775=ORIENTED_EDGE('',*,*,#7426,.F.);
#9776=ORIENTED_EDGE('',*,*,#7422,.F.);
#9777=ORIENTED_EDGE('',*,*,#7427,.F.);
#9778=ORIENTED_EDGE('',*,*,#7428,.F.);
#9779=ORIENTED_EDGE('',*,*,#7429,.F.);
#9780=ORIENTED_EDGE('',*,*,#7425,.F.);
#9781=ORIENTED_EDGE('',*,*,#7430,.F.);
#9782=ORIENTED_EDGE('',*,*,#7431,.T.);
#9783=ORIENTED_EDGE('',*,*,#7432,.F.);
#9784=ORIENTED_EDGE('',*,*,#7431,.F.);
#9785=ORIENTED_EDGE('',*,*,#7344,.T.);
#9786=ORIENTED_EDGE('',*,*,#7433,.T.);
#9787=ORIENTED_EDGE('',*,*,#7434,.T.);
#9788=ORIENTED_EDGE('',*,*,#7435,.F.);
#9789=ORIENTED_EDGE('',*,*,#7321,.T.);
#9790=ORIENTED_EDGE('',*,*,#7436,.F.);
#9791=ORIENTED_EDGE('',*,*,#7437,.F.);
#9792=ORIENTED_EDGE('',*,*,#7438,.T.);
#9793=ORIENTED_EDGE('',*,*,#7372,.T.);
#9794=ORIENTED_EDGE('',*,*,#7439,.T.);
#9795=ORIENTED_EDGE('',*,*,#7437,.T.);
#9796=ORIENTED_EDGE('',*,*,#7440,.F.);
#9797=ORIENTED_EDGE('',*,*,#7349,.T.);
#9798=ORIENTED_EDGE('',*,*,#7441,.F.);
#9799=ORIENTED_EDGE('',*,*,#7442,.F.);
#9800=ORIENTED_EDGE('',*,*,#7443,.T.);
#9801=ORIENTED_EDGE('',*,*,#7400,.T.);
#9802=ORIENTED_EDGE('',*,*,#7444,.T.);
#9803=ORIENTED_EDGE('',*,*,#7442,.T.);
#9804=ORIENTED_EDGE('',*,*,#7445,.F.);
#9805=ORIENTED_EDGE('',*,*,#7377,.T.);
#9806=ORIENTED_EDGE('',*,*,#7446,.F.);
#9807=ORIENTED_EDGE('',*,*,#7447,.F.);
#9808=ORIENTED_EDGE('',*,*,#7448,.T.);
#9809=ORIENTED_EDGE('',*,*,#7428,.T.);
#9810=ORIENTED_EDGE('',*,*,#7449,.T.);
#9811=ORIENTED_EDGE('',*,*,#7447,.T.);
#9812=ORIENTED_EDGE('',*,*,#7450,.F.);
#9813=ORIENTED_EDGE('',*,*,#7405,.T.);
#9814=ORIENTED_EDGE('',*,*,#7451,.F.);
#9815=ORIENTED_EDGE('',*,*,#7434,.F.);
#9816=ORIENTED_EDGE('',*,*,#7452,.T.);
#9817=ORIENTED_EDGE('',*,*,#7320,.T.);
#9818=ORIENTED_EDGE('',*,*,#7324,.T.);
#9819=ORIENTED_EDGE('',*,*,#7327,.T.);
#9820=ORIENTED_EDGE('',*,*,#7330,.T.);
#9821=ORIENTED_EDGE('',*,*,#7333,.T.);
#9822=ORIENTED_EDGE('',*,*,#7336,.T.);
#9823=ORIENTED_EDGE('',*,*,#7339,.T.);
#9824=ORIENTED_EDGE('',*,*,#7342,.T.);
#9825=ORIENTED_EDGE('',*,*,#7345,.T.);
#9826=ORIENTED_EDGE('',*,*,#7435,.T.);
#9827=ORIENTED_EDGE('',*,*,#7451,.T.);
#9828=ORIENTED_EDGE('',*,*,#7404,.T.);
#9829=ORIENTED_EDGE('',*,*,#7408,.T.);
#9830=ORIENTED_EDGE('',*,*,#7411,.T.);
#9831=ORIENTED_EDGE('',*,*,#7414,.T.);
#9832=ORIENTED_EDGE('',*,*,#7417,.T.);
#9833=ORIENTED_EDGE('',*,*,#7420,.T.);
#9834=ORIENTED_EDGE('',*,*,#7423,.T.);
#9835=ORIENTED_EDGE('',*,*,#7426,.T.);
#9836=ORIENTED_EDGE('',*,*,#7429,.T.);
#9837=ORIENTED_EDGE('',*,*,#7450,.T.);
#9838=ORIENTED_EDGE('',*,*,#7446,.T.);
#9839=ORIENTED_EDGE('',*,*,#7376,.T.);
#9840=ORIENTED_EDGE('',*,*,#7380,.T.);
#9841=ORIENTED_EDGE('',*,*,#7383,.T.);
#9842=ORIENTED_EDGE('',*,*,#7386,.T.);
#9843=ORIENTED_EDGE('',*,*,#7389,.T.);
#9844=ORIENTED_EDGE('',*,*,#7392,.T.);
#9845=ORIENTED_EDGE('',*,*,#7395,.T.);
#9846=ORIENTED_EDGE('',*,*,#7398,.T.);
#9847=ORIENTED_EDGE('',*,*,#7401,.T.);
#9848=ORIENTED_EDGE('',*,*,#7445,.T.);
#9849=ORIENTED_EDGE('',*,*,#7441,.T.);
#9850=ORIENTED_EDGE('',*,*,#7348,.T.);
#9851=ORIENTED_EDGE('',*,*,#7352,.T.);
#9852=ORIENTED_EDGE('',*,*,#7355,.T.);
#9853=ORIENTED_EDGE('',*,*,#7358,.T.);
#9854=ORIENTED_EDGE('',*,*,#7361,.T.);
#9855=ORIENTED_EDGE('',*,*,#7364,.T.);
#9856=ORIENTED_EDGE('',*,*,#7367,.T.);
#9857=ORIENTED_EDGE('',*,*,#7370,.T.);
#9858=ORIENTED_EDGE('',*,*,#7373,.T.);
#9859=ORIENTED_EDGE('',*,*,#7440,.T.);
#9860=ORIENTED_EDGE('',*,*,#7436,.T.);
#9861=ORIENTED_EDGE('',*,*,#7432,.T.);
#9862=ORIENTED_EDGE('',*,*,#7318,.T.);
#9863=ORIENTED_EDGE('',*,*,#7438,.F.);
#9864=ORIENTED_EDGE('',*,*,#7439,.F.);
#9865=ORIENTED_EDGE('',*,*,#7371,.T.);
#9866=ORIENTED_EDGE('',*,*,#7368,.T.);
#9867=ORIENTED_EDGE('',*,*,#7365,.T.);
#9868=ORIENTED_EDGE('',*,*,#7362,.T.);
#9869=ORIENTED_EDGE('',*,*,#7359,.T.);
#9870=ORIENTED_EDGE('',*,*,#7356,.T.);
#9871=ORIENTED_EDGE('',*,*,#7353,.T.);
#9872=ORIENTED_EDGE('',*,*,#7350,.T.);
#9873=ORIENTED_EDGE('',*,*,#7346,.T.);
#9874=ORIENTED_EDGE('',*,*,#7443,.F.);
#9875=ORIENTED_EDGE('',*,*,#7444,.F.);
#9876=ORIENTED_EDGE('',*,*,#7399,.T.);
#9877=ORIENTED_EDGE('',*,*,#7396,.T.);
#9878=ORIENTED_EDGE('',*,*,#7393,.T.);
#9879=ORIENTED_EDGE('',*,*,#7390,.T.);
#9880=ORIENTED_EDGE('',*,*,#7387,.T.);
#9881=ORIENTED_EDGE('',*,*,#7384,.T.);
#9882=ORIENTED_EDGE('',*,*,#7381,.T.);
#9883=ORIENTED_EDGE('',*,*,#7378,.T.);
#9884=ORIENTED_EDGE('',*,*,#7374,.T.);
#9885=ORIENTED_EDGE('',*,*,#7448,.F.);
#9886=ORIENTED_EDGE('',*,*,#7449,.F.);
#9887=ORIENTED_EDGE('',*,*,#7427,.T.);
#9888=ORIENTED_EDGE('',*,*,#7424,.T.);
#9889=ORIENTED_EDGE('',*,*,#7421,.T.);
#9890=ORIENTED_EDGE('',*,*,#7418,.T.);
#9891=ORIENTED_EDGE('',*,*,#7415,.T.);
#9892=ORIENTED_EDGE('',*,*,#7412,.T.);
#9893=ORIENTED_EDGE('',*,*,#7409,.T.);
#9894=ORIENTED_EDGE('',*,*,#7406,.T.);
#9895=ORIENTED_EDGE('',*,*,#7402,.T.);
#9896=ORIENTED_EDGE('',*,*,#7452,.F.);
#9897=ORIENTED_EDGE('',*,*,#7433,.F.);
#9898=ORIENTED_EDGE('',*,*,#7343,.T.);
#9899=ORIENTED_EDGE('',*,*,#7340,.T.);
#9900=ORIENTED_EDGE('',*,*,#7337,.T.);
#9901=ORIENTED_EDGE('',*,*,#7334,.T.);
#9902=ORIENTED_EDGE('',*,*,#7331,.T.);
#9903=ORIENTED_EDGE('',*,*,#7328,.T.);
#9904=ORIENTED_EDGE('',*,*,#7325,.T.);
#9905=ORIENTED_EDGE('',*,*,#7322,.T.);
#9906=ORIENTED_EDGE('',*,*,#7430,.T.);
#12073=CYLINDRICAL_SURFACE('',#14170,0.21);
#12539=ADVANCED_FACE('',(#1827),#1344,.F.);
#12540=ADVANCED_FACE('',(#1828),#1345,.F.);
#12541=ADVANCED_FACE('',(#1829),#1346,.F.);
#12542=ADVANCED_FACE('',(#1830),#1347,.F.);
#12543=ADVANCED_FACE('',(#1831),#1348,.F.);
#12544=ADVANCED_FACE('',(#1832),#1349,.F.);
#12545=ADVANCED_FACE('',(#1833),#1350,.F.);
#12546=ADVANCED_FACE('',(#1834),#1351,.F.);
#12547=ADVANCED_FACE('',(#1835),#1352,.F.);
#12548=ADVANCED_FACE('',(#1836),#1353,.F.);
#12549=ADVANCED_FACE('',(#1837),#1354,.F.);
#12550=ADVANCED_FACE('',(#1838),#1355,.F.);
#12551=ADVANCED_FACE('',(#1839),#1356,.F.);
#12552=ADVANCED_FACE('',(#1840),#1357,.F.);
#12553=ADVANCED_FACE('',(#1841),#1358,.F.);
#12554=ADVANCED_FACE('',(#1842),#1359,.F.);
#12555=ADVANCED_FACE('',(#1843),#1360,.F.);
#12556=ADVANCED_FACE('',(#1844),#1361,.F.);
#12557=ADVANCED_FACE('',(#1845),#1362,.F.);
#12558=ADVANCED_FACE('',(#1846),#1363,.F.);
#12559=ADVANCED_FACE('',(#1847),#1364,.F.);
#12560=ADVANCED_FACE('',(#1848),#1365,.F.);
#12561=ADVANCED_FACE('',(#1849),#1366,.F.);
#12562=ADVANCED_FACE('',(#1850),#1367,.F.);
#12563=ADVANCED_FACE('',(#1851),#1368,.F.);
#12564=ADVANCED_FACE('',(#1852),#1369,.F.);
#12565=ADVANCED_FACE('',(#1853),#1370,.F.);
#12566=ADVANCED_FACE('',(#1854),#1371,.F.);
#12567=ADVANCED_FACE('',(#1855),#1372,.F.);
#12568=ADVANCED_FACE('',(#1856),#1373,.F.);
#12569=ADVANCED_FACE('',(#1857),#1374,.F.);
#12570=ADVANCED_FACE('',(#1858),#1375,.F.);
#12571=ADVANCED_FACE('',(#1859),#1376,.F.);
#12572=ADVANCED_FACE('',(#1860),#1377,.F.);
#12573=ADVANCED_FACE('',(#1861),#1378,.F.);
#12574=ADVANCED_FACE('',(#1862),#1379,.F.);
#12575=ADVANCED_FACE('',(#1863),#12073,.F.);
#12576=ADVANCED_FACE('',(#1864),#1380,.T.);
#12577=ADVANCED_FACE('',(#1865),#1381,.T.);
#12578=ADVANCED_FACE('',(#1866),#1382,.T.);
#12579=ADVANCED_FACE('',(#1867),#1383,.T.);
#12580=ADVANCED_FACE('',(#1868),#1384,.T.);
#12581=ADVANCED_FACE('',(#1869),#1385,.T.);
#12582=ADVANCED_FACE('',(#1870),#1386,.T.);
#12583=ADVANCED_FACE('',(#1871),#1387,.T.);
#12584=ADVANCED_FACE('',(#1872,#1146),#1388,.T.);
#12585=ADVANCED_FACE('',(#1873,#1147),#1389,.F.);
#13044=CLOSED_SHELL('',(#12539,#12540,#12541,#12542,#12543,#12544,#12545,
#12546,#12547,#12548,#12549,#12550,#12551,#12552,#12553,#12554,#12555,#12556,
#12557,#12558,#12559,#12560,#12561,#12562,#12563,#12564,#12565,#12566,#12567,
#12568,#12569,#12570,#12571,#12572,#12573,#12574,#12575,#12576,#12577,#12578,
#12579,#12580,#12581,#12582,#12583,#12584,#12585));
#14133=AXIS2_PLACEMENT_3D('',#20377,#16291,#16292);
#14134=AXIS2_PLACEMENT_3D('',#20378,#16293,#16294);
#14135=AXIS2_PLACEMENT_3D('',#20387,#16299,#16300);
#14136=AXIS2_PLACEMENT_3D('',#20393,#16304,#16305);
#14137=AXIS2_PLACEMENT_3D('',#20399,#16309,#16310);
#14138=AXIS2_PLACEMENT_3D('',#20405,#16314,#16315);
#14139=AXIS2_PLACEMENT_3D('',#20411,#16319,#16320);
#14140=AXIS2_PLACEMENT_3D('',#20417,#16324,#16325);
#14141=AXIS2_PLACEMENT_3D('',#20423,#16329,#16330);
#14142=AXIS2_PLACEMENT_3D('',#20429,#16334,#16335);
#14143=AXIS2_PLACEMENT_3D('',#20435,#16339,#16340);
#14144=AXIS2_PLACEMENT_3D('',#20444,#16345,#16346);
#14145=AXIS2_PLACEMENT_3D('',#20450,#16350,#16351);
#14146=AXIS2_PLACEMENT_3D('',#20456,#16355,#16356);
#14147=AXIS2_PLACEMENT_3D('',#20462,#16360,#16361);
#14148=AXIS2_PLACEMENT_3D('',#20468,#16365,#16366);
#14149=AXIS2_PLACEMENT_3D('',#20474,#16370,#16371);
#14150=AXIS2_PLACEMENT_3D('',#20480,#16375,#16376);
#14151=AXIS2_PLACEMENT_3D('',#20486,#16380,#16381);
#14152=AXIS2_PLACEMENT_3D('',#20492,#16385,#16386);
#14153=AXIS2_PLACEMENT_3D('',#20501,#16391,#16392);
#14154=AXIS2_PLACEMENT_3D('',#20507,#16396,#16397);
#14155=AXIS2_PLACEMENT_3D('',#20513,#16401,#16402);
#14156=AXIS2_PLACEMENT_3D('',#20519,#16406,#16407);
#14157=AXIS2_PLACEMENT_3D('',#20525,#16411,#16412);
#14158=AXIS2_PLACEMENT_3D('',#20531,#16416,#16417);
#14159=AXIS2_PLACEMENT_3D('',#20537,#16421,#16422);
#14160=AXIS2_PLACEMENT_3D('',#20543,#16426,#16427);
#14161=AXIS2_PLACEMENT_3D('',#20549,#16431,#16432);
#14162=AXIS2_PLACEMENT_3D('',#20558,#16437,#16438);
#14163=AXIS2_PLACEMENT_3D('',#20564,#16442,#16443);
#14164=AXIS2_PLACEMENT_3D('',#20570,#16447,#16448);
#14165=AXIS2_PLACEMENT_3D('',#20576,#16452,#16453);
#14166=AXIS2_PLACEMENT_3D('',#20582,#16457,#16458);
#14167=AXIS2_PLACEMENT_3D('',#20588,#16462,#16463);
#14168=AXIS2_PLACEMENT_3D('',#20594,#16467,#16468);
#14169=AXIS2_PLACEMENT_3D('',#20600,#16472,#16473);
#14170=AXIS2_PLACEMENT_3D('',#20606,#16477,#16478);
#14171=AXIS2_PLACEMENT_3D('',#20608,#16479,#16480);
#14172=AXIS2_PLACEMENT_3D('',#20611,#16482,#16483);
#14173=AXIS2_PLACEMENT_3D('',#20612,#16484,#16485);
#14174=AXIS2_PLACEMENT_3D('',#20618,#16489,#16490);
#14175=AXIS2_PLACEMENT_3D('',#20624,#16494,#16495);
#14176=AXIS2_PLACEMENT_3D('',#20627,#16498,#16499);
#14177=AXIS2_PLACEMENT_3D('',#20633,#16503,#16504);
#14178=AXIS2_PLACEMENT_3D('',#20636,#16507,#16508);
#14179=AXIS2_PLACEMENT_3D('',#20642,#16512,#16513);
#14180=AXIS2_PLACEMENT_3D('',#20645,#16516,#16517);
#14181=AXIS2_PLACEMENT_3D('',#20648,#16520,#16521);
#14182=AXIS2_PLACEMENT_3D('',#20649,#16522,#16523);
#16291=DIRECTION('axis',(0.,0.,1.));
#16292=DIRECTION('refdir',(1.,0.,0.));
#16293=DIRECTION('center_axis',(0.,0.,-1.));
#16294=DIRECTION('ref_axis',(0.,1.,0.));
#16295=DIRECTION('',(0.,1.,0.));
#16296=DIRECTION('',(1.,0.,0.));
#16297=DIRECTION('',(0.,-1.,0.));
#16298=DIRECTION('',(1.,0.,0.));
#16299=DIRECTION('center_axis',(0.,1.,-8.88178419700125E-16));
#16300=DIRECTION('ref_axis',(0.,8.88178419700125E-16,1.));
#16301=DIRECTION('',(0.,8.88178419700125E-16,1.));
#16302=DIRECTION('',(1.,0.,0.));
#16303=DIRECTION('',(0.,-8.88178419700125E-16,-1.));
#16304=DIRECTION('center_axis',(0.,-7.40148683083439E-16,-1.));
#16305=DIRECTION('ref_axis',(0.,1.,-7.40148683083439E-16));
#16306=DIRECTION('',(0.,1.,-7.40148683083439E-16));
#16307=DIRECTION('',(1.,0.,0.));
#16308=DIRECTION('',(0.,-1.,7.40148683083439E-16));
#16309=DIRECTION('center_axis',(0.,-0.707106781186547,-0.707106781186548));
#16310=DIRECTION('ref_axis',(0.,0.707106781186548,-0.707106781186547));
#16311=DIRECTION('',(0.,0.707106781186548,-0.707106781186547));
#16312=DIRECTION('',(1.,0.,0.));
#16313=DIRECTION('',(0.,-0.707106781186548,0.707106781186547));
#16314=DIRECTION('center_axis',(0.,-1.,2.77555756156289E-16));
#16315=DIRECTION('ref_axis',(0.,-2.77555756156289E-16,-1.));
#16316=DIRECTION('',(0.,-2.77555756156289E-16,-1.));
#16317=DIRECTION('',(1.,0.,0.));
#16318=DIRECTION('',(0.,2.77555756156289E-16,1.));
#16319=DIRECTION('center_axis',(0.,-0.707106781186547,0.707106781186548));
#16320=DIRECTION('ref_axis',(0.,-0.707106781186548,-0.707106781186547));
#16321=DIRECTION('',(0.,-0.707106781186548,-0.707106781186547));
#16322=DIRECTION('',(1.,0.,0.));
#16323=DIRECTION('',(0.,0.707106781186548,0.707106781186547));
#16324=DIRECTION('center_axis',(0.,7.40148683083438E-16,1.));
#16325=DIRECTION('ref_axis',(0.,-1.,7.40148683083438E-16));
#16326=DIRECTION('',(0.,-1.,7.40148683083438E-16));
#16327=DIRECTION('',(1.,0.,0.));
#16328=DIRECTION('',(0.,1.,-7.40148683083438E-16));
#16329=DIRECTION('center_axis',(0.,1.,-4.44089209850063E-16));
#16330=DIRECTION('ref_axis',(0.,4.44089209850063E-16,1.));
#16331=DIRECTION('',(0.,4.44089209850063E-16,1.));
#16332=DIRECTION('',(1.,0.,0.));
#16333=DIRECTION('',(0.,-4.44089209850063E-16,-1.));
#16334=DIRECTION('center_axis',(0.,2.41352831440251E-16,1.));
#16335=DIRECTION('ref_axis',(0.,-1.,2.41352831440251E-16));
#16336=DIRECTION('',(0.,-1.,2.41352831440251E-16));
#16337=DIRECTION('',(-1.,0.,0.));
#16338=DIRECTION('',(0.,1.,-2.41352831440251E-16));
#16339=DIRECTION('center_axis',(0.,-1.,2.41352831440251E-16));
#16340=DIRECTION('ref_axis',(0.,-2.41352831440251E-16,-1.));
#16341=DIRECTION('',(0.,-2.41352831440251E-16,-1.));
#16342=DIRECTION('',(1.,0.,0.));
#16343=DIRECTION('',(0.,2.41352831440251E-16,1.));
#16344=DIRECTION('',(1.,0.,0.));
#16345=DIRECTION('center_axis',(0.,0.,-1.));
#16346=DIRECTION('ref_axis',(0.,1.,0.));
#16347=DIRECTION('',(0.,1.,0.));
#16348=DIRECTION('',(1.,0.,0.));
#16349=DIRECTION('',(0.,-1.,0.));
#16350=DIRECTION('center_axis',(0.,-1.,0.));
#16351=DIRECTION('ref_axis',(0.,0.,-1.));
#16352=DIRECTION('',(0.,0.,-1.));
#16353=DIRECTION('',(1.,0.,0.));
#16354=DIRECTION('',(0.,0.,1.));
#16355=DIRECTION('center_axis',(0.,-0.707106781186547,0.707106781186548));
#16356=DIRECTION('ref_axis',(0.,-0.707106781186548,-0.707106781186547));
#16357=DIRECTION('',(0.,-0.707106781186548,-0.707106781186547));
#16358=DIRECTION('',(1.,0.,0.));
#16359=DIRECTION('',(0.,0.707106781186548,0.707106781186547));
#16360=DIRECTION('center_axis',(0.,0.,1.));
#16361=DIRECTION('ref_axis',(0.,-1.,0.));
#16362=DIRECTION('',(0.,-1.,0.));
#16363=DIRECTION('',(1.,0.,0.));
#16364=DIRECTION('',(0.,1.,0.));
#16365=DIRECTION('center_axis',(0.,0.707106781186548,0.707106781186547));
#16366=DIRECTION('ref_axis',(0.,-0.707106781186547,0.707106781186548));
#16367=DIRECTION('',(0.,-0.707106781186547,0.707106781186548));
#16368=DIRECTION('',(1.,0.,0.));
#16369=DIRECTION('',(0.,0.707106781186547,-0.707106781186548));
#16370=DIRECTION('center_axis',(0.,1.,0.));
#16371=DIRECTION('ref_axis',(0.,0.,1.));
#16372=DIRECTION('',(0.,0.,1.));
#16373=DIRECTION('',(1.,0.,0.));
#16374=DIRECTION('',(0.,0.,-1.));
#16375=DIRECTION('center_axis',(0.,0.,-1.));
#16376=DIRECTION('ref_axis',(0.,1.,0.));
#16377=DIRECTION('',(0.,1.,0.));
#16378=DIRECTION('',(1.,0.,0.));
#16379=DIRECTION('',(0.,-1.,0.));
#16380=DIRECTION('center_axis',(0.,1.,-2.41352831440251E-16));
#16381=DIRECTION('ref_axis',(0.,2.41352831440251E-16,1.));
#16382=DIRECTION('',(0.,2.41352831440251E-16,1.));
#16383=DIRECTION('',(-1.,0.,0.));
#16384=DIRECTION('',(0.,-2.41352831440251E-16,-1.));
#16385=DIRECTION('center_axis',(0.,0.,1.));
#16386=DIRECTION('ref_axis',(0.,-1.,0.));
#16387=DIRECTION('',(0.,-1.,0.));
#16388=DIRECTION('',(1.,0.,0.));
#16389=DIRECTION('',(0.,1.,0.));
#16390=DIRECTION('',(1.,0.,0.));
#16391=DIRECTION('center_axis',(0.,-1.,0.));
#16392=DIRECTION('ref_axis',(0.,0.,-1.));
#16393=DIRECTION('',(0.,0.,-1.));
#16394=DIRECTION('',(1.,0.,0.));
#16395=DIRECTION('',(0.,0.,1.));
#16396=DIRECTION('center_axis',(0.,0.,1.));
#16397=DIRECTION('ref_axis',(0.,-1.,0.));
#16398=DIRECTION('',(0.,-1.,0.));
#16399=DIRECTION('',(1.,0.,0.));
#16400=DIRECTION('',(0.,1.,0.));
#16401=DIRECTION('center_axis',(0.,0.707106781186548,0.707106781186548));
#16402=DIRECTION('ref_axis',(0.,-0.707106781186548,0.707106781186548));
#16403=DIRECTION('',(0.,-0.707106781186548,0.707106781186548));
#16404=DIRECTION('',(1.,0.,0.));
#16405=DIRECTION('',(0.,0.707106781186548,-0.707106781186548));
#16406=DIRECTION('center_axis',(0.,1.,0.));
#16407=DIRECTION('ref_axis',(0.,0.,1.));
#16408=DIRECTION('',(0.,0.,1.));
#16409=DIRECTION('',(1.,0.,0.));
#16410=DIRECTION('',(0.,0.,-1.));
#16411=DIRECTION('center_axis',(0.,0.707106781186548,-0.707106781186547));
#16412=DIRECTION('ref_axis',(0.,0.707106781186547,0.707106781186548));
#16413=DIRECTION('',(0.,0.707106781186547,0.707106781186548));
#16414=DIRECTION('',(1.,0.,0.));
#16415=DIRECTION('',(0.,-0.707106781186547,-0.707106781186548));
#16416=DIRECTION('center_axis',(0.,-7.40148683083438E-16,-1.));
#16417=DIRECTION('ref_axis',(0.,1.,-7.40148683083438E-16));
#16418=DIRECTION('',(0.,1.,-7.40148683083438E-16));
#16419=DIRECTION('',(1.,0.,0.));
#16420=DIRECTION('',(0.,-1.,7.40148683083438E-16));
#16421=DIRECTION('center_axis',(0.,-1.,0.));
#16422=DIRECTION('ref_axis',(0.,0.,-1.));
#16423=DIRECTION('',(0.,0.,-1.));
#16424=DIRECTION('',(1.,0.,0.));
#16425=DIRECTION('',(0.,0.,1.));
#16426=DIRECTION('center_axis',(0.,0.,-1.));
#16427=DIRECTION('ref_axis',(0.,1.,0.));
#16428=DIRECTION('',(0.,1.,0.));
#16429=DIRECTION('',(-1.,0.,0.));
#16430=DIRECTION('',(0.,-1.,0.));
#16431=DIRECTION('center_axis',(0.,1.,0.));
#16432=DIRECTION('ref_axis',(0.,0.,1.));
#16433=DIRECTION('',(0.,0.,1.));
#16434=DIRECTION('',(1.,0.,0.));
#16435=DIRECTION('',(0.,0.,-1.));
#16436=DIRECTION('',(1.,0.,0.));
#16437=DIRECTION('center_axis',(0.,0.,1.));
#16438=DIRECTION('ref_axis',(0.,-1.,0.));
#16439=DIRECTION('',(0.,-1.,0.));
#16440=DIRECTION('',(1.,0.,0.));
#16441=DIRECTION('',(0.,1.,0.));
#16442=DIRECTION('center_axis',(0.,1.,0.));
#16443=DIRECTION('ref_axis',(0.,0.,1.));
#16444=DIRECTION('',(0.,0.,1.));
#16445=DIRECTION('',(1.,0.,0.));
#16446=DIRECTION('',(0.,0.,-1.));
#16447=DIRECTION('center_axis',(0.,0.707106781186547,-0.707106781186548));
#16448=DIRECTION('ref_axis',(0.,0.707106781186548,0.707106781186547));
#16449=DIRECTION('',(0.,0.707106781186548,0.707106781186547));
#16450=DIRECTION('',(1.,0.,0.));
#16451=DIRECTION('',(0.,-0.707106781186548,-0.707106781186547));
#16452=DIRECTION('center_axis',(0.,0.,-1.));
#16453=DIRECTION('ref_axis',(0.,1.,0.));
#16454=DIRECTION('',(0.,1.,0.));
#16455=DIRECTION('',(1.,0.,0.));
#16456=DIRECTION('',(0.,-1.,0.));
#16457=DIRECTION('center_axis',(0.,-0.707106781186547,-0.707106781186548));
#16458=DIRECTION('ref_axis',(0.,0.707106781186548,-0.707106781186547));
#16459=DIRECTION('',(0.,0.707106781186548,-0.707106781186547));
#16460=DIRECTION('',(1.,0.,0.));
#16461=DIRECTION('',(0.,-0.707106781186548,0.707106781186547));
#16462=DIRECTION('center_axis',(0.,-1.,0.));
#16463=DIRECTION('ref_axis',(0.,0.,-1.));
#16464=DIRECTION('',(0.,0.,-1.));
#16465=DIRECTION('',(1.,0.,0.));
#16466=DIRECTION('',(0.,0.,1.));
#16467=DIRECTION('center_axis',(0.,0.,1.));
#16468=DIRECTION('ref_axis',(0.,-1.,0.));
#16469=DIRECTION('',(0.,-1.,0.));
#16470=DIRECTION('',(1.,0.,0.));
#16471=DIRECTION('',(0.,1.,0.));
#16472=DIRECTION('center_axis',(0.,-1.,0.));
#16473=DIRECTION('ref_axis',(0.,0.,-1.));
#16474=DIRECTION('',(0.,0.,-1.));
#16475=DIRECTION('',(-1.,0.,0.));
#16476=DIRECTION('',(0.,0.,1.));
#16477=DIRECTION('center_axis',(1.,0.,0.));
#16478=DIRECTION('ref_axis',(0.,0.,-1.));
#16479=DIRECTION('center_axis',(1.,0.,0.));
#16480=DIRECTION('ref_axis',(0.,0.,-1.));
#16481=DIRECTION('',(1.,0.,0.));
#16482=DIRECTION('center_axis',(-1.,0.,0.));
#16483=DIRECTION('ref_axis',(0.,0.,-1.));
#16484=DIRECTION('center_axis',(0.,1.,0.));
#16485=DIRECTION('ref_axis',(0.,0.,1.));
#16486=DIRECTION('',(0.,0.,1.));
#16487=DIRECTION('',(1.,0.,0.));
#16488=DIRECTION('',(0.,0.,1.));
#16489=DIRECTION('center_axis',(0.,1.,0.));
#16490=DIRECTION('ref_axis',(0.,0.,1.));
#16491=DIRECTION('',(0.,0.,1.));
#16492=DIRECTION('',(1.,0.,0.));
#16493=DIRECTION('',(0.,0.,1.));
#16494=DIRECTION('center_axis',(0.,0.,-1.));
#16495=DIRECTION('ref_axis',(0.,1.,0.));
#16496=DIRECTION('',(0.,1.,0.));
#16497=DIRECTION('',(0.,1.,0.));
#16498=DIRECTION('center_axis',(0.,0.,-1.));
#16499=DIRECTION('ref_axis',(0.,1.,0.));
#16500=DIRECTION('',(0.,1.,0.));
#16501=DIRECTION('',(1.,0.,0.));
#16502=DIRECTION('',(0.,1.,0.));
#16503=DIRECTION('center_axis',(0.,-1.,0.));
#16504=DIRECTION('ref_axis',(0.,0.,-1.));
#16505=DIRECTION('',(0.,0.,-1.));
#16506=DIRECTION('',(0.,0.,-1.));
#16507=DIRECTION('center_axis',(0.,-1.,0.));
#16508=DIRECTION('ref_axis',(0.,0.,-1.));
#16509=DIRECTION('',(0.,0.,-1.));
#16510=DIRECTION('',(1.,0.,0.));
#16511=DIRECTION('',(0.,0.,-1.));
#16512=DIRECTION('center_axis',(0.,0.,1.));
#16513=DIRECTION('ref_axis',(0.,-1.,0.));
#16514=DIRECTION('',(0.,-1.,0.));
#16515=DIRECTION('',(0.,-1.,0.));
#16516=DIRECTION('center_axis',(0.,0.,1.));
#16517=DIRECTION('ref_axis',(0.,-1.,0.));
#16518=DIRECTION('',(0.,-1.,0.));
#16519=DIRECTION('',(0.,-1.,0.));
#16520=DIRECTION('center_axis',(1.,0.,0.));
#16521=DIRECTION('ref_axis',(0.,0.,-1.));
#16522=DIRECTION('center_axis',(1.,0.,0.));
#16523=DIRECTION('ref_axis',(0.,0.,-1.));
#20377=CARTESIAN_POINT('',(0.,0.,0.));
#20378=CARTESIAN_POINT('Origin',(-0.1,0.82,-0.3));
#20379=CARTESIAN_POINT('',(-1.,0.82,-0.3));
#20380=CARTESIAN_POINT('',(-1.,1.,-0.3));
#20381=CARTESIAN_POINT('',(-1.,0.41,-0.3));
#20382=CARTESIAN_POINT('',(30.,0.82,-0.3));
#20383=CARTESIAN_POINT('',(-0.1,0.82,-0.3));
#20384=CARTESIAN_POINT('',(30.,1.,-0.3));
#20385=CARTESIAN_POINT('',(30.,0.41,-0.3));
#20386=CARTESIAN_POINT('',(-0.05,1.,-0.3));
#20387=CARTESIAN_POINT('Origin',(-0.1,0.82,-0.55));
#20388=CARTESIAN_POINT('',(-1.,0.82,-0.55));
#20389=CARTESIAN_POINT('',(-1.,0.82,-0.275));
#20390=CARTESIAN_POINT('',(30.,0.82,-0.55));
#20391=CARTESIAN_POINT('',(-0.1,0.82,-0.55));
#20392=CARTESIAN_POINT('',(30.,0.82,-0.275));
#20393=CARTESIAN_POINT('Origin',(-0.1,0.67,-0.55));
#20394=CARTESIAN_POINT('',(-1.,0.67,-0.55));
#20395=CARTESIAN_POINT('',(-1.,0.335,-0.55));
#20396=CARTESIAN_POINT('',(30.,0.67,-0.55));
#20397=CARTESIAN_POINT('',(-0.1,0.67,-0.55));
#20398=CARTESIAN_POINT('',(30.,0.335,-0.55));
#20399=CARTESIAN_POINT('Origin',(-0.1,0.42,-0.3));
#20400=CARTESIAN_POINT('',(-1.,0.42,-0.3));
#20401=CARTESIAN_POINT('',(-1.,0.24,-0.12));
#20402=CARTESIAN_POINT('',(30.,0.42,-0.3));
#20403=CARTESIAN_POINT('',(-0.1,0.42,-0.3));
#20404=CARTESIAN_POINT('',(30.,0.24,-0.12));
#20405=CARTESIAN_POINT('Origin',(-0.1,0.42,0.3));
#20406=CARTESIAN_POINT('',(-1.,0.42,0.3));
#20407=CARTESIAN_POINT('',(-1.,0.42,0.15));
#20408=CARTESIAN_POINT('',(30.,0.42,0.3));
#20409=CARTESIAN_POINT('',(-0.1,0.42,0.3));
#20410=CARTESIAN_POINT('',(30.,0.42,0.15));
#20411=CARTESIAN_POINT('Origin',(-0.1,0.67,0.55));
#20412=CARTESIAN_POINT('',(-1.,0.67,0.55));
#20413=CARTESIAN_POINT('',(-1.,0.365,0.245));
#20414=CARTESIAN_POINT('',(30.,0.67,0.55));
#20415=CARTESIAN_POINT('',(-0.1,0.67,0.55));
#20416=CARTESIAN_POINT('',(30.,0.365,0.245));
#20417=CARTESIAN_POINT('Origin',(-0.1,0.82,0.55));
#20418=CARTESIAN_POINT('',(-1.,0.82,0.55));
#20419=CARTESIAN_POINT('',(-1.,0.41,0.55));
#20420=CARTESIAN_POINT('',(30.,0.82,0.55));
#20421=CARTESIAN_POINT('',(-0.1,0.82,0.55));
#20422=CARTESIAN_POINT('',(30.,0.41,0.55));
#20423=CARTESIAN_POINT('Origin',(-0.1,0.82,0.3));
#20424=CARTESIAN_POINT('',(-1.,0.82,0.3));
#20425=CARTESIAN_POINT('',(-1.,0.82,0.15));
#20426=CARTESIAN_POINT('',(30.,0.82,0.3));
#20427=CARTESIAN_POINT('',(-0.1,0.82,0.3));
#20428=CARTESIAN_POINT('',(30.,0.82,0.15));
#20429=CARTESIAN_POINT('Origin',(-0.1,1.05,0.3));
#20430=CARTESIAN_POINT('',(-1.,1.,0.3));
#20431=CARTESIAN_POINT('',(-1.,0.525,0.3));
#20432=CARTESIAN_POINT('',(30.,1.,0.3));
#20433=CARTESIAN_POINT('',(-0.05,1.,0.3));
#20434=CARTESIAN_POINT('',(30.,0.525,0.3));
#20435=CARTESIAN_POINT('Origin',(-0.1,-0.3,-0.82));
#20436=CARTESIAN_POINT('',(-1.,-0.3,-0.82));
#20437=CARTESIAN_POINT('',(-1.,-0.3,-1.));
#20438=CARTESIAN_POINT('',(-1.,-0.3,-0.41));
#20439=CARTESIAN_POINT('',(30.,-0.3,-0.82));
#20440=CARTESIAN_POINT('',(-0.1,-0.3,-0.82));
#20441=CARTESIAN_POINT('',(30.,-0.3,-1.));
#20442=CARTESIAN_POINT('',(30.,-0.3,-0.41));
#20443=CARTESIAN_POINT('',(-0.05,-0.3,-1.));
#20444=CARTESIAN_POINT('Origin',(-0.1,-0.55,-0.82));
#20445=CARTESIAN_POINT('',(-1.,-0.55,-0.82));
#20446=CARTESIAN_POINT('',(-1.,-0.275,-0.82));
#20447=CARTESIAN_POINT('',(30.,-0.55,-0.82));
#20448=CARTESIAN_POINT('',(-0.1,-0.55,-0.82));
#20449=CARTESIAN_POINT('',(30.,-0.275,-0.82));
#20450=CARTESIAN_POINT('Origin',(-0.1,-0.55,-0.67));
#20451=CARTESIAN_POINT('',(-1.,-0.55,-0.67));
#20452=CARTESIAN_POINT('',(-1.,-0.55,-0.335));
#20453=CARTESIAN_POINT('',(30.,-0.55,-0.67));
#20454=CARTESIAN_POINT('',(-0.1,-0.55,-0.67));
#20455=CARTESIAN_POINT('',(30.,-0.55,-0.335));
#20456=CARTESIAN_POINT('Origin',(-0.1,-0.3,-0.42));
#20457=CARTESIAN_POINT('',(-1.,-0.3,-0.42));
#20458=CARTESIAN_POINT('',(-1.,-0.12,-0.24));
#20459=CARTESIAN_POINT('',(30.,-0.3,-0.42));
#20460=CARTESIAN_POINT('',(-0.1,-0.3,-0.42));
#20461=CARTESIAN_POINT('',(30.,-0.12,-0.24));
#20462=CARTESIAN_POINT('Origin',(-0.1,0.3,-0.42));
#20463=CARTESIAN_POINT('',(-1.,0.3,-0.42));
#20464=CARTESIAN_POINT('',(-1.,0.15,-0.42));
#20465=CARTESIAN_POINT('',(30.,0.3,-0.42));
#20466=CARTESIAN_POINT('',(-0.1,0.3,-0.42));
#20467=CARTESIAN_POINT('',(30.,0.15,-0.42));
#20468=CARTESIAN_POINT('Origin',(-0.1,0.55,-0.67));
#20469=CARTESIAN_POINT('',(-1.,0.55,-0.67));
#20470=CARTESIAN_POINT('',(-1.,0.245,-0.365));
#20471=CARTESIAN_POINT('',(30.,0.55,-0.67));
#20472=CARTESIAN_POINT('',(-0.1,0.55,-0.67));
#20473=CARTESIAN_POINT('',(30.,0.245,-0.365));
#20474=CARTESIAN_POINT('Origin',(-0.1,0.55,-0.82));
#20475=CARTESIAN_POINT('',(-1.,0.55,-0.82));
#20476=CARTESIAN_POINT('',(-1.,0.55,-0.41));
#20477=CARTESIAN_POINT('',(30.,0.55,-0.82));
#20478=CARTESIAN_POINT('',(-0.1,0.55,-0.82));
#20479=CARTESIAN_POINT('',(30.,0.55,-0.41));
#20480=CARTESIAN_POINT('Origin',(-0.1,0.3,-0.82));
#20481=CARTESIAN_POINT('',(-1.,0.3,-0.82));
#20482=CARTESIAN_POINT('',(-1.,0.15,-0.82));
#20483=CARTESIAN_POINT('',(30.,0.3,-0.82));
#20484=CARTESIAN_POINT('',(-0.1,0.3,-0.82));
#20485=CARTESIAN_POINT('',(30.,0.15,-0.82));
#20486=CARTESIAN_POINT('Origin',(-0.1,0.3,-1.05));
#20487=CARTESIAN_POINT('',(-1.,0.3,-1.));
#20488=CARTESIAN_POINT('',(-1.,0.3,-0.525));
#20489=CARTESIAN_POINT('',(30.,0.3,-1.));
#20490=CARTESIAN_POINT('',(-0.05,0.3,-1.));
#20491=CARTESIAN_POINT('',(30.,0.3,-0.525));
#20492=CARTESIAN_POINT('Origin',(-0.1,-0.82,0.3));
#20493=CARTESIAN_POINT('',(-1.,-0.82,0.3));
#20494=CARTESIAN_POINT('',(-1.,-1.,0.3));
#20495=CARTESIAN_POINT('',(-1.,-0.41,0.3));
#20496=CARTESIAN_POINT('',(30.,-0.82,0.3));
#20497=CARTESIAN_POINT('',(-0.1,-0.82,0.3));
#20498=CARTESIAN_POINT('',(30.,-1.,0.3));
#20499=CARTESIAN_POINT('',(30.,-0.41,0.3));
#20500=CARTESIAN_POINT('',(-0.05,-1.,0.3));
#20501=CARTESIAN_POINT('Origin',(-0.1,-0.82,0.55));
#20502=CARTESIAN_POINT('',(-1.,-0.82,0.55));
#20503=CARTESIAN_POINT('',(-1.,-0.82,0.275));
#20504=CARTESIAN_POINT('',(30.,-0.82,0.55));
#20505=CARTESIAN_POINT('',(-0.1,-0.82,0.55));
#20506=CARTESIAN_POINT('',(30.,-0.82,0.275));
#20507=CARTESIAN_POINT('Origin',(-0.1,-0.67,0.55));
#20508=CARTESIAN_POINT('',(-1.,-0.67,0.55));
#20509=CARTESIAN_POINT('',(-1.,-0.335,0.55));
#20510=CARTESIAN_POINT('',(30.,-0.67,0.55));
#20511=CARTESIAN_POINT('',(-0.1,-0.67,0.55));
#20512=CARTESIAN_POINT('',(30.,-0.335,0.55));
#20513=CARTESIAN_POINT('Origin',(-0.1,-0.42,0.3));
#20514=CARTESIAN_POINT('',(-1.,-0.42,0.3));
#20515=CARTESIAN_POINT('',(-1.,-0.24,0.12));
#20516=CARTESIAN_POINT('',(30.,-0.42,0.3));
#20517=CARTESIAN_POINT('',(-0.1,-0.42,0.3));
#20518=CARTESIAN_POINT('',(30.,-0.24,0.12));
#20519=CARTESIAN_POINT('Origin',(-0.1,-0.42,-0.3));
#20520=CARTESIAN_POINT('',(-1.,-0.42,-0.3));
#20521=CARTESIAN_POINT('',(-1.,-0.42,-0.15));
#20522=CARTESIAN_POINT('',(30.,-0.42,-0.3));
#20523=CARTESIAN_POINT('',(-0.1,-0.42,-0.3));
#20524=CARTESIAN_POINT('',(30.,-0.42,-0.15));
#20525=CARTESIAN_POINT('Origin',(-0.1,-0.67,-0.55));
#20526=CARTESIAN_POINT('',(-1.,-0.67,-0.55));
#20527=CARTESIAN_POINT('',(-1.,-0.365,-0.245));
#20528=CARTESIAN_POINT('',(30.,-0.67,-0.55));
#20529=CARTESIAN_POINT('',(-0.1,-0.67,-0.55));
#20530=CARTESIAN_POINT('',(30.,-0.365,-0.245));
#20531=CARTESIAN_POINT('Origin',(-0.1,-0.82,-0.55));
#20532=CARTESIAN_POINT('',(-1.,-0.82,-0.55));
#20533=CARTESIAN_POINT('',(-1.,-0.41,-0.55));
#20534=CARTESIAN_POINT('',(30.,-0.82,-0.55));
#20535=CARTESIAN_POINT('',(-0.1,-0.82,-0.55));
#20536=CARTESIAN_POINT('',(30.,-0.41,-0.55));
#20537=CARTESIAN_POINT('Origin',(-0.1,-0.82,-0.3));
#20538=CARTESIAN_POINT('',(-1.,-0.82,-0.3));
#20539=CARTESIAN_POINT('',(-1.,-0.82,-0.15));
#20540=CARTESIAN_POINT('',(30.,-0.82,-0.3));
#20541=CARTESIAN_POINT('',(-0.1,-0.82,-0.3));
#20542=CARTESIAN_POINT('',(30.,-0.82,-0.15));
#20543=CARTESIAN_POINT('Origin',(-0.1,-1.05,-0.3));
#20544=CARTESIAN_POINT('',(-1.,-1.,-0.3));
#20545=CARTESIAN_POINT('',(-1.,-0.525,-0.3));
#20546=CARTESIAN_POINT('',(30.,-1.,-0.3));
#20547=CARTESIAN_POINT('',(-0.05,-1.,-0.3));
#20548=CARTESIAN_POINT('',(30.,-0.525,-0.3));
#20549=CARTESIAN_POINT('Origin',(-0.1,0.3,0.82));
#20550=CARTESIAN_POINT('',(-1.,0.3,0.82));
#20551=CARTESIAN_POINT('',(-1.,0.3,1.));
#20552=CARTESIAN_POINT('',(-1.,0.3,0.41));
#20553=CARTESIAN_POINT('',(30.,0.3,0.82));
#20554=CARTESIAN_POINT('',(-0.1,0.3,0.82));
#20555=CARTESIAN_POINT('',(30.,0.3,1.));
#20556=CARTESIAN_POINT('',(30.,0.3,0.41));
#20557=CARTESIAN_POINT('',(-0.05,0.3,1.));
#20558=CARTESIAN_POINT('Origin',(-0.1,0.55,0.82));
#20559=CARTESIAN_POINT('',(-1.,0.55,0.82));
#20560=CARTESIAN_POINT('',(-1.,0.275,0.82));
#20561=CARTESIAN_POINT('',(30.,0.55,0.82));
#20562=CARTESIAN_POINT('',(-0.1,0.55,0.82));
#20563=CARTESIAN_POINT('',(30.,0.275,0.82));
#20564=CARTESIAN_POINT('Origin',(-0.1,0.55,0.67));
#20565=CARTESIAN_POINT('',(-1.,0.55,0.67));
#20566=CARTESIAN_POINT('',(-1.,0.55,0.335));
#20567=CARTESIAN_POINT('',(30.,0.55,0.67));
#20568=CARTESIAN_POINT('',(-0.1,0.55,0.67));
#20569=CARTESIAN_POINT('',(30.,0.55,0.335));
#20570=CARTESIAN_POINT('Origin',(-0.1,0.3,0.42));
#20571=CARTESIAN_POINT('',(-1.,0.3,0.42));
#20572=CARTESIAN_POINT('',(-1.,0.12,0.24));
#20573=CARTESIAN_POINT('',(30.,0.3,0.42));
#20574=CARTESIAN_POINT('',(-0.1,0.3,0.42));
#20575=CARTESIAN_POINT('',(30.,0.12,0.24));
#20576=CARTESIAN_POINT('Origin',(-0.1,-0.3,0.42));
#20577=CARTESIAN_POINT('',(-1.,-0.3,0.42));
#20578=CARTESIAN_POINT('',(-1.,-0.15,0.42));
#20579=CARTESIAN_POINT('',(30.,-0.3,0.42));
#20580=CARTESIAN_POINT('',(-0.1,-0.3,0.42));
#20581=CARTESIAN_POINT('',(30.,-0.15,0.42));
#20582=CARTESIAN_POINT('Origin',(-0.1,-0.55,0.67));
#20583=CARTESIAN_POINT('',(-1.,-0.55,0.67));
#20584=CARTESIAN_POINT('',(-1.,-0.245,0.365));
#20585=CARTESIAN_POINT('',(30.,-0.55,0.67));
#20586=CARTESIAN_POINT('',(-0.1,-0.55,0.67));
#20587=CARTESIAN_POINT('',(30.,-0.245,0.365));
#20588=CARTESIAN_POINT('Origin',(-0.1,-0.55,0.82));
#20589=CARTESIAN_POINT('',(-1.,-0.55,0.82));
#20590=CARTESIAN_POINT('',(-1.,-0.55,0.41));
#20591=CARTESIAN_POINT('',(30.,-0.55,0.82));
#20592=CARTESIAN_POINT('',(-0.1,-0.55,0.82));
#20593=CARTESIAN_POINT('',(30.,-0.55,0.41));
#20594=CARTESIAN_POINT('Origin',(-0.1,-0.3,0.82));
#20595=CARTESIAN_POINT('',(-1.,-0.3,0.82));
#20596=CARTESIAN_POINT('',(-1.,-0.15,0.82));
#20597=CARTESIAN_POINT('',(30.,-0.3,0.82));
#20598=CARTESIAN_POINT('',(-0.1,-0.3,0.82));
#20599=CARTESIAN_POINT('',(30.,-0.15,0.82));
#20600=CARTESIAN_POINT('Origin',(-0.1,-0.3,1.05));
#20601=CARTESIAN_POINT('',(-1.,-0.3,1.));
#20602=CARTESIAN_POINT('',(-1.,-0.3,0.525));
#20603=CARTESIAN_POINT('',(30.,-0.3,1.));
#20604=CARTESIAN_POINT('',(-0.05,-0.3,1.));
#20605=CARTESIAN_POINT('',(30.,-0.3,0.525));
#20606=CARTESIAN_POINT('Origin',(-0.1,0.,0.));
#20607=CARTESIAN_POINT('',(-1.,-2.57175827820944E-17,0.21));
#20608=CARTESIAN_POINT('Origin',(-1.,0.,0.));
#20609=CARTESIAN_POINT('',(30.,2.57175827820944E-17,0.21));
#20610=CARTESIAN_POINT('',(-0.1,-2.57175827820944E-17,0.21));
#20611=CARTESIAN_POINT('Origin',(30.,0.,0.));
#20612=CARTESIAN_POINT('Origin',(0.,1.,-1.));
#20613=CARTESIAN_POINT('',(-1.,1.,1.));
#20614=CARTESIAN_POINT('',(-1.,1.,-0.5));
#20615=CARTESIAN_POINT('',(30.,1.,1.));
#20616=CARTESIAN_POINT('',(0.,1.,1.));
#20617=CARTESIAN_POINT('',(30.,1.,-1.));
#20618=CARTESIAN_POINT('Origin',(0.,1.,-1.));
#20619=CARTESIAN_POINT('',(30.,1.,-1.));
#20620=CARTESIAN_POINT('',(30.,1.,-1.));
#20621=CARTESIAN_POINT('',(-1.,1.,-1.));
#20622=CARTESIAN_POINT('',(0.,1.,-1.));
#20623=CARTESIAN_POINT('',(-1.,1.,-0.5));
#20624=CARTESIAN_POINT('Origin',(0.,-1.,-1.));
#20625=CARTESIAN_POINT('',(-1.,-0.5,-1.));
#20626=CARTESIAN_POINT('',(30.,-1.,-1.));
#20627=CARTESIAN_POINT('Origin',(0.,-1.,-1.));
#20628=CARTESIAN_POINT('',(30.,-1.,-1.));
#20629=CARTESIAN_POINT('',(30.,-1.,-1.));
#20630=CARTESIAN_POINT('',(-1.,-1.,-1.));
#20631=CARTESIAN_POINT('',(0.,-1.,-1.));
#20632=CARTESIAN_POINT('',(-1.,-0.5,-1.));
#20633=CARTESIAN_POINT('Origin',(0.,-1.,1.));
#20634=CARTESIAN_POINT('',(-1.,-1.,0.5));
#20635=CARTESIAN_POINT('',(30.,-1.,1.));
#20636=CARTESIAN_POINT('Origin',(0.,-1.,1.));
#20637=CARTESIAN_POINT('',(30.,-1.,1.));
#20638=CARTESIAN_POINT('',(30.,-1.,1.));
#20639=CARTESIAN_POINT('',(-1.,-1.,1.));
#20640=CARTESIAN_POINT('',(0.,-1.,1.));
#20641=CARTESIAN_POINT('',(-1.,-1.,0.5));
#20642=CARTESIAN_POINT('Origin',(0.,1.,1.));
#20643=CARTESIAN_POINT('',(-1.,0.5,1.));
#20644=CARTESIAN_POINT('',(30.,1.,1.));
#20645=CARTESIAN_POINT('Origin',(0.,1.,1.));
#20646=CARTESIAN_POINT('',(30.,1.,1.));
#20647=CARTESIAN_POINT('',(-1.,0.5,1.));
#20648=CARTESIAN_POINT('Origin',(30.,0.,0.));
#20649=CARTESIAN_POINT('Origin',(-1.,0.,0.));
#33901=UNCERTAINTY_MEASURE_WITH_UNIT(LENGTH_MEASURE(0.001),#33982,
'DISTANCE_ACCURACY_VALUE',
'Maximum model space distance between geometric entities at asserted c
onnectivities');
#33929=UNCERTAINTY_MEASURE_WITH_UNIT(LENGTH_MEASURE(0.001),#33982,
'DISTANCE_ACCURACY_VALUE',
'Maximum model space distance between geometric entities at asserted c
onnectivities');
#33953=(
GEOMETRIC_REPRESENTATION_CONTEXT(3)
GLOBAL_UNCERTAINTY_ASSIGNED_CONTEXT((#33901))
GLOBAL_UNIT_ASSIGNED_CONTEXT((#33982,#33984,#33985))
REPRESENTATION_CONTEXT('','3D')
);
#33981=(
GEOMETRIC_REPRESENTATION_CONTEXT(3)
GLOBAL_UNCERTAINTY_ASSIGNED_CONTEXT((#33929))
GLOBAL_UNIT_ASSIGNED_CONTEXT((#33982,#33984,#33985))
REPRESENTATION_CONTEXT('','3D')
);
#33982=(
LENGTH_UNIT()
NAMED_UNIT(*)
SI_UNIT(.CENTI.,.METRE.)
);
#33984=(
NAMED_UNIT(*)
PLANE_ANGLE_UNIT()
SI_UNIT($,.RADIAN.)
);
#33985=(
NAMED_UNIT(*)
SI_UNIT($,.STERADIAN.)
SOLID_ANGLE_UNIT()
);
#34009=SHAPE_DEFINITION_REPRESENTATION(#34070,#34205);
#34070=PRODUCT_DEFINITION_SHAPE('',$,#34257);
#34205=SHAPE_REPRESENTATION('',(#14133),#33953);
#34233=PRODUCT_DEFINITION_CONTEXT('part definition',#34388,'design');
#34257=PRODUCT_DEFINITION('Slotted Extrusion - 20 x 20 x 300 mm',
'Slotted Extrusion - 20 x 20 x 300 mm',#34308,#34233);
#34308=PRODUCT_DEFINITION_FORMATION('',$,#34413);
#34388=APPLICATION_CONTEXT(
'Core Data for Automotive Mechanical Design Process');
#34389=PRODUCT_CONTEXT('part definition',#34388,'mechanical');
#34413=PRODUCT('Slotted Extrusion - 20 x 20 x 300 mm',
'Slotted Extrusion - 20 x 20 x 300 mm',
'Slotted Extrusion - 20 x 20 x 300 mm',(#34389));
#34525=COLOUR_RGB('Off White',0.89,0.88,0.83);
#34526=FILL_AREA_STYLE_COLOUR('',#34525);
#34527=FILL_AREA_STYLE('',(#34526));
#34528=SURFACE_STYLE_FILL_AREA(#34527);
#34529=SURFACE_SIDE_STYLE('',(#34528));
#34530=SURFACE_STYLE_USAGE(.BOTH.,#34529);
#34531=PRESENTATION_STYLE_ASSIGNMENT((#34530));
ENDSEC;
END-ISO-10303-21;
